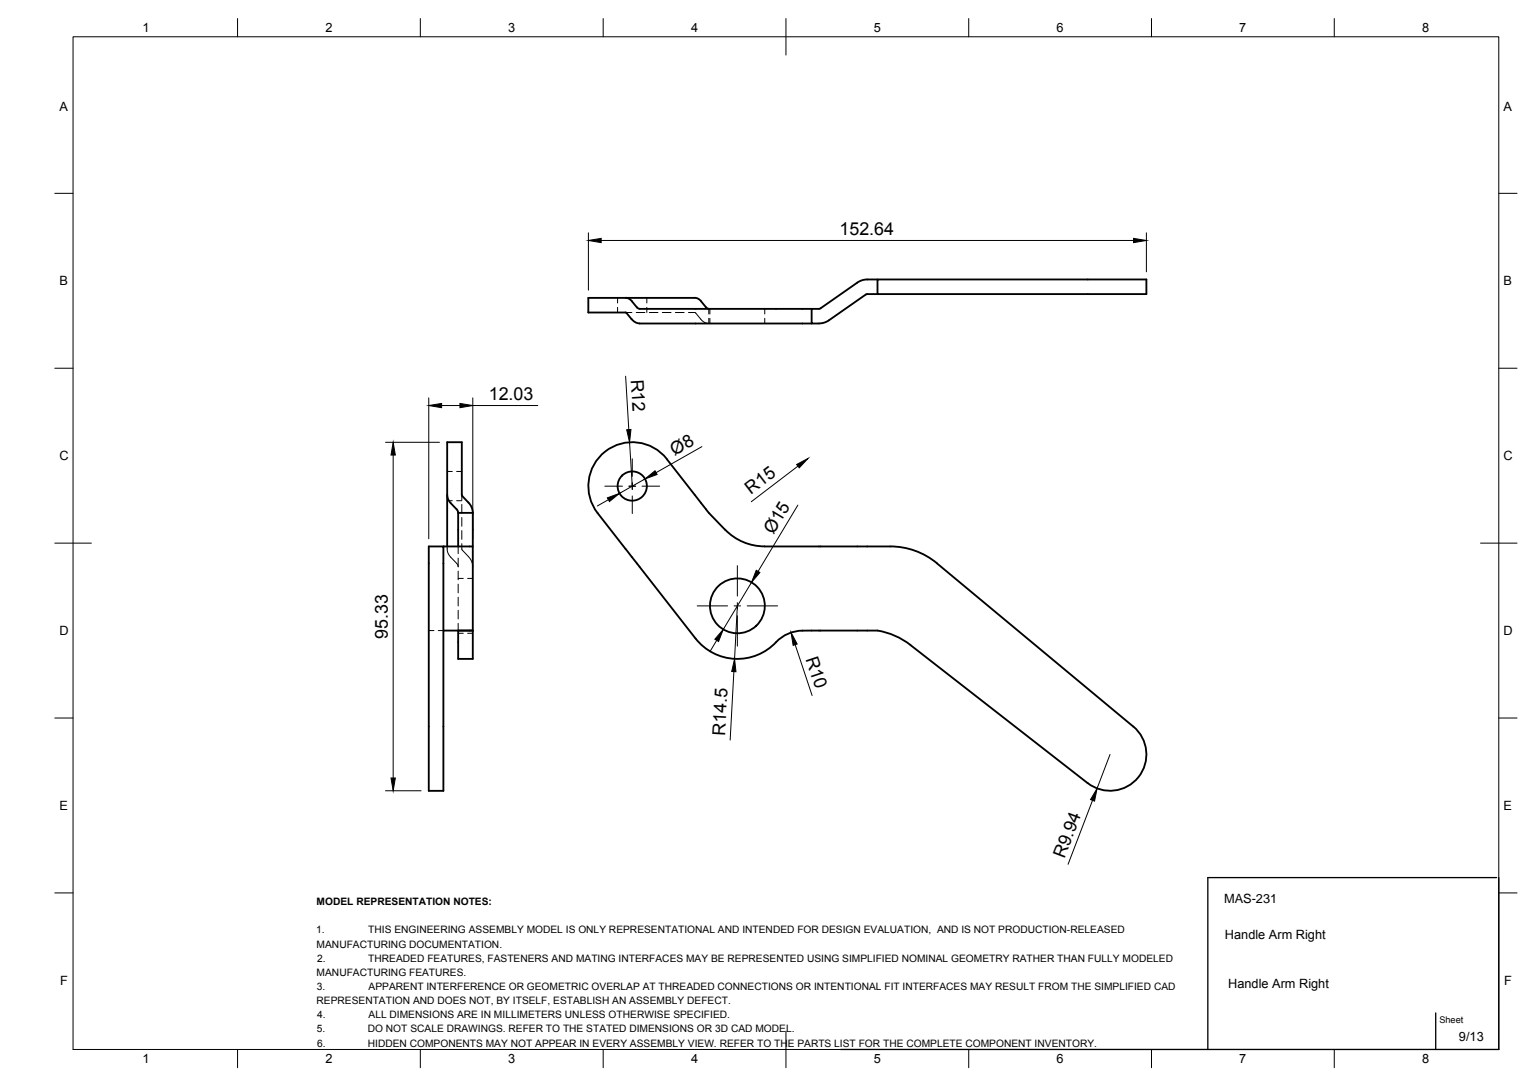
ISO-10303-21;
HEADER;
FILE_DESCRIPTION (('STEP AP214'),
    '1' );
FILE_NAME ( 'Handle Arm Right.step', '2026-10-04T02:08:54', ( '' ), ( '' ), 'STEP AP214', 'Unspecified', '' );
FILE_SCHEMA (( 'AUTOMOTIVE_DESIGN' ));
ENDSEC;
DATA;
#96=CARTESIAN_POINT ( 'NONE',  ( 0.3108999017613323090, 0.9251089822459528378, -1.060267534067256046 ) ) ;
#148=DIRECTION ( 'NONE',  ( -1.000000000000000000, 0.000000000000000000, 0.000000000000000000 ) ) ;
#150=ORIENTED_EDGE ( 'NONE', *, *, #2837, .F. ) ;
#154=DIRECTION ( 'NONE',  ( -1.000000000000000000, -1.802250327717385127E-14, 1.473544972410982106E-14 ) ) ;
#160=DIRECTION ( 'NONE',  ( 0.8191520442889949072, -0.4519843998600416302, 0.3531289150159167556 ) ) ;
#183=VERTEX_POINT ( 'NONE', #42256 ) ;
#188=VECTOR ( 'NONE', #38666, 39.37007874015748143 ) ;
#232=CARTESIAN_POINT ( 'NONE',  ( 0.3161444924769701292, 2.177585298233984279, -3.731703755406948986 ) ) ;
#267=VECTOR ( 'NONE', #18707, 39.37007874015748143 ) ;
#305=CARTESIAN_POINT ( 'NONE',  ( 0.1574803149606299191, 0.5360961046428496246, -0.7563373642699310340 ) ) ;
#307=AXIS2_PLACEMENT_3D ( 'NONE', #8881, #45755, #23738 ) ;
#333=DIRECTION ( 'NONE',  ( 1.000000000000000000, 2.891205793294678326E-16, 0.000000000000000000 ) ) ;
#432=FILL_AREA_STYLE_COLOUR ( '', #44690 ) ;
#457=CARTESIAN_POINT ( 'NONE',  ( 0.2759478392031653460, -0.09842519685039370636, 2.185526306663015728 ) ) ;
#475=DIRECTION ( 'NONE',  ( 0.5735764363510417185, 0.6455006197386566891, -0.5043203561029927506 ) ) ;
#563=CARTESIAN_POINT ( 'NONE',  ( 0.2759478392031586291, -3.539702385322740129E-16, 1.224299699984019663 ) ) ;
#580=VERTEX_POINT ( 'NONE', #5172 ) ;
#606=CARTESIAN_POINT ( 'NONE',  ( 0.1574803149606299191, 0.6241017553149685870, 0.3240160679609070948 ) ) ;
#622=CYLINDRICAL_SURFACE ( 'NONE', #2285, 0.1574803149606297803 ) ;
#656=DIRECTION ( 'NONE',  ( -1.000000000000000000, 0.000000000000000000, 7.051687499798870116E-15 ) ) ;
#688=ORIENTED_EDGE ( 'NONE', *, *, #3021, .T. ) ;
#710=ORIENTED_EDGE ( 'NONE', *, *, #12023, .T. ) ;
#712=VERTEX_POINT ( 'NONE', #45900 ) ;
#730=ADVANCED_FACE ( 'NONE', ( #7834 ), #25829, .F. ) ;
#732=DIRECTION ( 'NONE',  ( 0.000000000000000000, -0.7880107536067199048, 0.6156614753256609562 ) ) ;
#801=CARTESIAN_POINT ( 'NONE',  ( 0.1627249056762492263, 1.099487083487564965, -0.04739565599252298922 ) ) ;
#842=DIRECTION ( 'NONE',  ( 0.7986355100472960489, 0.000000000000000000, -0.6018150231520441595 ) ) ;
#890=ORIENTED_EDGE ( 'NONE', *, *, #19656, .T. ) ;
#907=DIRECTION ( 'NONE',  ( 0.8191520442889899112, -0.4519843998600478474, 0.3531289150159199197 ) ) ;
#943=DIRECTION ( 'NONE',  ( -0.8191520442889950182, 0.4519843998600410750, -0.3531289150159169776 ) ) ;
#974=CIRCLE ( 'NONE', #3327, 0.5708661417322835607 ) ;
#1013=CYLINDRICAL_SURFACE ( 'NONE', #11687, 0.1574803149606297803 ) ;
#1016=CARTESIAN_POINT ( 'NONE',  ( 0.3161444924769291065, 1.914733266569315084, -0.6843357808987579061 ) ) ;
#1036=AXIS2_PLACEMENT_3D ( 'NONE', #44067, #21807, #46957 ) ;
#1075=EDGE_CURVE ( 'NONE', #17962, #28784, #34674, .T. ) ;
#1118=AXIS2_PLACEMENT_3D ( 'NONE', #47069, #18320, #21680 ) ;
#1213=CARTESIAN_POINT ( 'NONE',  ( 0.1574803149606299191, 0.4668427075568346574, -0.7022306805398661478 ) ) ;
#1249=CARTESIAN_POINT ( 'NONE',  ( 0.1574803149606299191, 0.5288907983920094757, -0.7507079620615707549 ) ) ;
#1265=PLANE ( 'NONE',  #18594 ) ;
#1322=FACE_OUTER_BOUND ( 'NONE', #41297, .T. ) ;
#1360=CIRCLE ( 'NONE', #22783, 0.2362204724409449064 ) ;
#1386=CARTESIAN_POINT ( 'NONE',  ( 0.1184675242425283492, -0.5708661417322835607, 1.214596435718460654 ) ) ;
#1400=VECTOR ( 'NONE', #475, 39.37007874015748143 ) ;
#1404=ORIENTED_EDGE ( 'NONE', *, *, #13116, .F. ) ;
#1526=CARTESIAN_POINT ( 'NONE',  ( 0.000000000000000000, 0.6305768042517894134, -0.4926605935704669315 ) ) ;
#1542=LINE ( 'NONE', #23135, #39059 ) ;
#1655=ORIENTED_EDGE ( 'NONE', *, *, #10241, .T. ) ;
#1671=VECTOR ( 'NONE', #1986, 39.37007874015748854 ) ;
#1698=FACE_OUTER_BOUND ( 'NONE', #16346, .T. ) ;
#1743=DIRECTION ( 'NONE',  ( 7.155734338404322954E-15, 0.000000000000000000, 1.000000000000000000 ) ) ;
#1767=VERTEX_POINT ( 'NONE', #2534 ) ;
#1780=VECTOR ( 'NONE', #20781, 39.37007874015748143 ) ;
#1820=DIRECTION ( 'NONE',  ( -5.724375810226263558E-16, -0.6156614753256592909, -0.7880107536067213481 ) ) ;
#1831=CARTESIAN_POINT ( 'NONE',  ( 0.1574803149606299191, 0.3740157480314960647, 1.004692544842683111 ) ) ;
#1839=ORIENTED_EDGE ( 'NONE', *, *, #26366, .T. ) ;
#1843=LINE ( 'NONE', #23903, #35866 ) ;
#1867=ORIENTED_EDGE ( 'NONE', *, *, #8153, .F. ) ;
#1870=CARTESIAN_POINT ( 'NONE',  ( 0.1574803149606299191, 0.4668427075568346574, -0.7022306805398661478 ) ) ;
#1872=DIRECTION ( 'NONE',  ( 1.000000000000000000, 0.000000000000000000, 0.000000000000000000 ) ) ;
#1903=ADVANCED_FACE ( 'NONE', ( #8262 ), #36341, .T. ) ;
#1912=LINE ( 'NONE', #35237, #37906 ) ;
#1986=DIRECTION ( 'NONE',  ( 0.000000000000000000, 0.7880107536067212370, -0.6156614753256591799 ) ) ;
#1997=CARTESIAN_POINT ( 'NONE',  ( 0.4736248074375440931, 1.890321945096787193, -4.194630839571732217 ) ) ;
#2053=CARTESIAN_POINT ( 'NONE',  ( 0.000000000000000000, 0.4666052258408008302, -0.7025346432751023995 ) ) ;
#2057=VERTEX_POINT ( 'NONE', #16188 ) ;
#2085=ORIENTED_EDGE ( 'NONE', *, *, #38033, .T. ) ;
#2127=ORIENTED_EDGE ( 'NONE', *, *, #36636, .T. ) ;
#2131=CYLINDRICAL_SURFACE ( 'NONE', #6486, 0.3912448816427545051 ) ;
#2137=CYLINDRICAL_SURFACE ( 'NONE', #29140, 0.07874015748031498729 ) ;
#2139=CARTESIAN_POINT ( 'NONE',  ( 0.1574803149606299191, 1.086379535891623949, -0.03715491745706125948 ) ) ;
#2146=EDGE_CURVE ( 'NONE', #36896, #18734, #9944, .T. ) ;
#2162=EDGE_CURVE ( 'NONE', #18566, #33555, #16421, .T. ) ;
#2164=DIRECTION ( 'NONE',  ( 7.051687499798870116E-15, 0.000000000000000000, 1.000000000000000000 ) ) ;
#2197=VERTEX_POINT ( 'NONE', #4657 ) ;
#2230=AXIS2_PLACEMENT_3D ( 'NONE', #33648, #41237, #4840 ) ;
#2255=DIRECTION ( 'NONE',  ( 1.109243974507663983E-29, 1.000000000000000000, 2.355041373848515369E-15 ) ) ;
#2285=AXIS2_PLACEMENT_3D ( 'NONE', #44710, #29474, #29932 ) ;
#2368=VECTOR ( 'NONE', #43957, 39.37007874015748854 ) ;
#2426=DIRECTION ( 'NONE',  ( 5.724375810226264544E-16, 0.6156614753256587358, 0.7880107536067215701 ) ) ;
#2515=CARTESIAN_POINT ( 'NONE',  ( 0.3161444924769165610, 1.798092712879858279, -3.826876940038417718 ) ) ;
#2525=AXIS2_PLACEMENT_3D ( 'NONE', #19014, #29636, #37478 ) ;
#2534=CARTESIAN_POINT ( 'NONE',  ( 0.1574803149606299191, 0.4666052258408008302, -0.7025346432751023995 ) ) ;
#2537=ORIENTED_EDGE ( 'NONE', *, *, #20684, .T. ) ;
#2566=DIRECTION ( 'NONE',  ( -3.769839275579535403E-17, 0.7880107536067207930, -0.6156614753256599570 ) ) ;
#2570=CARTESIAN_POINT ( 'NONE',  ( 0.3161444924769519216, 1.488499961090669288, -0.3513258257898460579 ) ) ;
#2588=ORIENTED_EDGE ( 'NONE', *, *, #47395, .F. ) ;
#2603=MECHANICAL_DESIGN_GEOMETRIC_PRESENTATION_REPRESENTATION('',(#12604),#30958);
#2604=DIRECTION ( 'NONE',  ( 1.000000000000000000, 0.000000000000000000, 0.000000000000000000 ) ) ;
#2675=DIRECTION ( 'NONE',  ( -1.000000000000000000, 5.464378949326940770E-15, -4.275490733183370330E-15 ) ) ;
#2683=VECTOR ( 'NONE', #9528, 39.37007874015748854 ) ;
#2700=CARTESIAN_POINT ( 'NONE',  ( 0.4399002236966062518, 0.8539303365987028771, -1.004656681308842447 ) ) ;
#2715=ORIENTED_EDGE ( 'NONE', *, *, #40441, .T. ) ;
#2761=ORIENTED_EDGE ( 'NONE', *, *, #28717, .F. ) ;
#2806=DIRECTION ( 'NONE',  ( 0.000000000000000000, -0.7880107536067206819, 0.6156614753256598460 ) ) ;
#2831=CARTESIAN_POINT ( 'NONE',  ( 0.1126279540338996077, -0.5708661417322835607, 1.206847064312610129 ) ) ;
#2837=EDGE_CURVE ( 'NONE', #24150, #15113, #31611, .T. ) ;
#2918=CARTESIAN_POINT ( 'NONE',  ( 0.3161444924769535869, 1.690605217543005745, -0.5092277576975102749 ) ) ;
#2936=UNCERTAINTY_MEASURE_WITH_UNIT (LENGTH_MEASURE( 1.000000000000000082E-05 ), #19423, 'distance_accuracy_value', 'NONE') ;
#2944=EDGE_LOOP ( 'NONE', ( #31065, #44061, #24696, #6082 ) ) ;
#2955=LINE ( 'NONE', #43213, #5714 ) ;
#2989=EDGE_LOOP ( 'NONE', ( #22664, #46106, #42101, #21732 ) ) ;
#3005=CIRCLE ( 'NONE', #2230, 0.2362204724409449064 ) ;
#3021=EDGE_CURVE ( 'NONE', #7776, #30501, #22148, .T. ) ;
#3044=ORIENTED_EDGE ( 'NONE', *, *, #24684, .T. ) ;
#3053=EDGE_CURVE ( 'NONE', #36104, #36896, #36781, .T. ) ;
#3055=EDGE_LOOP ( 'NONE', ( #8748, #27707, #12776, #33393, #5370, #22939, #8609, #37631, #5677, #29321, #36750, #3117 ) ) ;
#3117=ORIENTED_EDGE ( 'NONE', *, *, #33699, .F. ) ;
#3135=ORIENTED_EDGE ( 'NONE', *, *, #11426, .T. ) ;
#3173=ORIENTED_EDGE ( 'NONE', *, *, #15768, .T. ) ;
#3241=ORIENTED_EDGE ( 'NONE', *, *, #7301, .T. ) ;
#3327=AXIS2_PLACEMENT_3D ( 'NONE', #20136, #12966, #17479 ) ;
#3369=ORIENTED_EDGE ( 'NONE', *, *, #29054, .T. ) ;
#3463=CARTESIAN_POINT ( 'NONE',  ( 0.2759478392031617933, -0.09842519685039370636, 1.713085361781127913 ) ) ;
#3493=CIRCLE ( 'NONE', #30313, 0.3937007874015747699 ) ;
#3515=DIRECTION ( 'NONE',  ( 0.000000000000000000, 2.355041373848520102E-15, -1.000000000000000000 ) ) ;
#3551=CARTESIAN_POINT ( 'NONE',  ( 0.1184675242425281411, 0.3740157480314960647, 1.224299699984021661 ) ) ;
#3566=CARTESIAN_POINT ( 'NONE',  ( 0.2442368959035201015, -0.5708661417322835607, 1.119822416324439018 ) ) ;
#3572=ORIENTED_EDGE ( 'NONE', *, *, #45147, .T. ) ;
#3575=ADVANCED_FACE ( 'NONE', ( #38939 ), #43233, .F. ) ;
#3706=AXIS2_PLACEMENT_3D ( 'NONE', #42837, #2604, #10047 ) ;
#3797=AXIS2_PLACEMENT_3D ( 'NONE', #37657, #19436, #732 ) ;
#3803=CARTESIAN_POINT ( 'NONE',  ( 0.1184675242425198838, 0.000000000000000000, -8.353959598330964227E-16 ) ) ;
#3820=FACE_OUTER_BOUND ( 'NONE', #2989, .T. ) ;
#3827=DIRECTION ( 'NONE',  ( 0.000000000000000000, -1.000000000000000000, 0.000000000000000000 ) ) ;
#3830=ORIENTED_EDGE ( 'NONE', *, *, #41683, .T. ) ;
#3851=EDGE_LOOP ( 'NONE', ( #30997, #24195, #8872, #24931 ) ) ;
#3866=AXIS2_PLACEMENT_3D ( 'NONE', #19137, #5003, #15329 ) ;
#3913=DIRECTION ( 'NONE',  ( -5.159318851433039196E-16, -0.6156614753256609562, -0.7880107536067197938 ) ) ;
#3919=ADVANCED_FACE ( 'NONE', ( #25099 ), #31607, .T. ) ;
#3923=DIRECTION ( 'NONE',  ( -2.114720919224289611E-16, 1.000000000000000000, 0.000000000000000000 ) ) ;
#3930=VECTOR ( 'NONE', #23402, 39.37007874015748143 ) ;
#3971=APPLICATION_CONTEXT ( 'automotive_design' ) ;
#3980=LINE ( 'NONE', #606, #11849 ) ;
#4054=DIRECTION ( 'NONE',  ( 7.047314121155781188E-15, 0.000000000000000000, 1.000000000000000000 ) ) ;
#4143=DIRECTION ( 'NONE',  ( -1.000000000000000000, 0.000000000000000000, -7.051687499798870116E-15 ) ) ;
#4164=DIRECTION ( 'NONE',  ( -5.298843091159153171E-15, -2.355041373848512214E-15, 1.000000000000000000 ) ) ;
#4180=VERTEX_POINT ( 'NONE', #43155 ) ;
#4190=VECTOR ( 'NONE', #3913, 39.37007874015748143 ) ;
#4197=ORIENTED_EDGE ( 'NONE', *, *, #32553, .F. ) ;
#4223=CARTESIAN_POINT ( 'NONE',  ( 0.02847999302535491814, 0.6072747502901004735, -0.8119482170283445210 ) ) ;
#4250=EDGE_CURVE ( 'NONE', #712, #6130, #37711, .T. ) ;
#4273=CARTESIAN_POINT ( 'NONE',  ( 0.4736248074375630224, 0.4457451269443653552, -1.671447902550338815 ) ) ;
#4317=CARTESIAN_POINT ( 'NONE',  ( 0.1864803149606299171, 1.086379535891623949, -0.03715491745706173132 ) ) ;
#4384=DIRECTION ( 'NONE',  ( 0.000000000000000000, -0.6156614753256598460, -0.7880107536067206819 ) ) ;
#4416=ORIENTED_EDGE ( 'NONE', *, *, #40562, .F. ) ;
#4445=EDGE_LOOP ( 'NONE', ( #3241, #15111, #25556, #32618 ) ) ;
#4448=PLANE ( 'NONE',  #30350 ) ;
#4454=EDGE_LOOP ( 'NONE', ( #30362, #10226, #35204, #29981 ) ) ;
#4469=DIRECTION ( 'NONE',  ( -1.000000000000000000, 0.000000000000000000, 0.000000000000000000 ) ) ;
#4470=EDGE_CURVE ( 'NONE', #32150, #42931, #18249, .T. ) ;
#4527=VECTOR ( 'NONE', #17737, 39.37007874015748143 ) ;
#4531=EDGE_LOOP ( 'NONE', ( #18099, #28878, #35700, #13225 ) ) ;
#4543=EDGE_CURVE ( 'NONE', #27121, #2057, #46998, .T. ) ;
#4625=CARTESIAN_POINT ( 'NONE',  ( 0.1184675242425078795, -0.09842519685039370636, 1.713085361781127913 ) ) ;
#4657=CARTESIAN_POINT ( 'NONE',  ( 2.048885995248196921E-16, -0.5708661417322835607, 0.9783464566929134243 ) ) ;
#4663=DIRECTION ( 'NONE',  ( -4.275490733183370330E-15, 0.000000000000000000, 1.000000000000000000 ) ) ;
#4725=CARTESIAN_POINT ( 'NONE',  ( 0.000000000000000000, 3.616083068348484413E-17, -0.2952755905511810774 ) ) ;
#4741=LINE ( 'NONE', #33791, #6344 ) ;
#4755=AXIS2_PLACEMENT_3D ( 'NONE', #5649, #20260, #6102 ) ;
#4767=ORIENTED_EDGE ( 'NONE', *, *, #18776, .T. ) ;
#4840=DIRECTION ( 'NONE',  ( 1.000000000000000000, 2.891205793294678326E-16, 0.000000000000000000 ) ) ;
#4880=MANIFOLD_SOLID_BREP ( 'Handle Arm Right', #31751 ) ;
#4924=PLANE ( 'NONE',  #29481 ) ;
#4948=AXIS2_PLACEMENT_3D ( 'NONE', #23717, #5496, #30694 ) ;
#4958=CARTESIAN_POINT ( 'NONE',  ( 0.2759478392031653460, 0.3740157480314960647, 2.185526306663015728 ) ) ;
#4972=ADVANCED_FACE ( 'NONE', ( #36875, #11476 ), #40211, .T. ) ;
#5003=DIRECTION ( 'NONE',  ( 5.724375810226257641E-16, 0.6156614753256588468, 0.7880107536067216811 ) ) ;
#5082=FACE_OUTER_BOUND ( 'NONE', #14954, .T. ) ;
#5117=ORIENTED_EDGE ( 'NONE', *, *, #23549, .T. ) ;
#5144=CARTESIAN_POINT ( 'NONE',  ( 0.1184675242425078795, -0.09842519685039370636, 1.713085361781127913 ) ) ;
#5172=CARTESIAN_POINT ( 'NONE',  ( 0.4736248074375835060, 1.690605217543005745, -0.5092277576975118292 ) ) ;
#5237=DIRECTION ( 'NONE',  ( -5.464378949326941559E-15, -1.000000000000000000, 0.000000000000000000 ) ) ;
#5247=ORIENTED_EDGE ( 'NONE', *, *, #4250, .T. ) ;
#5343=CARTESIAN_POINT ( 'NONE',  ( 0.03372458374097370148, 0.6131769916352027838, -0.8165595533554468322 ) ) ;
#5367=CARTESIAN_POINT ( 'NONE',  ( 0.1733357866104494327, -0.5708661417322835607, 1.025733466389925352 ) ) ;
#5370=ORIENTED_EDGE ( 'NONE', *, *, #44949, .F. ) ;
#5378=FACE_OUTER_BOUND ( 'NONE', #29897, .T. ) ;
#5401=AXIS2_PLACEMENT_3D ( 'NONE', #42962, #13754, #6791 ) ;
#5403=CARTESIAN_POINT ( 'NONE',  ( 0.4736248074375433714, 2.559880088878740079, -3.648497683167389649 ) ) ;
#5446=VECTOR ( 'NONE', #41680, 39.37007874015748143 ) ;
#5465=DIRECTION ( 'NONE',  ( -1.000000000000000000, -1.413024824309076326E-14, 1.884033099078770012E-14 ) ) ;
#5479=CIRCLE ( 'NONE', #39127, 0.3912448816427545051 ) ;
#5496=DIRECTION ( 'NONE',  ( 4.190354514309263844E-15, -0.9699617890481126992, -0.2432573283306889433 ) ) ;
#5536=ADVANCED_BREP_SHAPE_REPRESENTATION ( 'Handle Arm Right', ( #4880, #20860 ), #27025 ) ;
#5540=DIRECTION ( 'NONE',  ( 0.000000000000000000, 2.355041373848520102E-15, -1.000000000000000000 ) ) ;
#5563=FACE_OUTER_BOUND ( 'NONE', #13406, .T. ) ;
#5570=ADVANCED_FACE ( 'NONE', ( #20635, #41946 ), #39074, .F. ) ;
#5584=DIRECTION ( 'NONE',  ( -1.000000000000000000, 0.000000000000000000, 7.155734338404321376E-15 ) ) ;
#5625=CIRCLE ( 'NONE', #2525, 0.4724409448818896462 ) ;
#5626=VERTEX_POINT ( 'NONE', #28572 ) ;
#5649=CARTESIAN_POINT ( 'NONE',  ( 0.1864803149606299171, 1.086379535891623949, -0.03715491745706165500 ) ) ;
#5673=ORIENTED_EDGE ( 'NONE', *, *, #42018, .F. ) ;
#5677=ORIENTED_EDGE ( 'NONE', *, *, #17755, .F. ) ;
#5708=PLANE ( 'NONE',  #6732 ) ;
#5714=VECTOR ( 'NONE', #13761, 39.37007874015748854 ) ;
#5748=ADVANCED_FACE ( 'NONE', ( #11772 ), #37375, .T. ) ;
#5862=EDGE_CURVE ( 'NONE', #18361, #8850, #42608, .T. ) ;
#5864=VERTEX_POINT ( 'NONE', #2139 ) ;
#5962=AXIS2_PLACEMENT_3D ( 'NONE', #40068, #25952, #17812 ) ;
#5964=CARTESIAN_POINT ( 'NONE',  ( 0.2362204724409449064, -0.5708661417322835607, 0.9783464566929134243 ) ) ;
#5979=CIRCLE ( 'NONE', #45788, 0.4724409448818899238 ) ;
#6019=CARTESIAN_POINT ( 'NONE',  ( 0.2871444924769520068, 1.495705267341507883, -0.3569552279982047271 ) ) ;
#6035=DIRECTION ( 'NONE',  ( 0.000000000000000000, -1.000000000000000000, 0.000000000000000000 ) ) ;
#6082=ORIENTED_EDGE ( 'NONE', *, *, #34470, .F. ) ;
#6102=DIRECTION ( 'NONE',  ( -0.8191520442889957954, 0.4519843998600397428, -0.3531289150159173662 ) ) ;
#6130=VERTEX_POINT ( 'NONE', #25072 ) ;
#6254=ORIENTED_EDGE ( 'NONE', *, *, #27428, .T. ) ;
#6306=VERTEX_POINT ( 'NONE', #33949 ) ;
#6324=DIRECTION ( 'NONE',  ( -1.000000000000000000, 0.000000000000000000, 0.000000000000000000 ) ) ;
#6326=ADVANCED_FACE ( 'NONE', ( #20474 ), #13302, .T. ) ;
#6344=VECTOR ( 'NONE', #907, 39.37007874015748854 ) ;
#6404=DIRECTION ( 'NONE',  ( -1.000000000000000000, 0.000000000000000000, 0.000000000000000000 ) ) ;
#6428=EDGE_CURVE ( 'NONE', #11697, #44566, #23137, .T. ) ;
#6464=CARTESIAN_POINT ( 'NONE',  ( 0.1627249056762490320, 0.5419983459879528231, -0.7609487005970335671 ) ) ;
#6486=AXIS2_PLACEMENT_3D ( 'NONE', #16302, #30930, #31162 ) ;
#6525=ORIENTED_EDGE ( 'NONE', *, *, #8153, .T. ) ;
#6535=FACE_OUTER_BOUND ( 'NONE', #33407, .T. ) ;
#6567=AXIS2_PLACEMENT_3D ( 'NONE', #25527, #6324, #31990 ) ;
#6621=ORIENTED_EDGE ( 'NONE', *, *, #38033, .F. ) ;
#6626=CARTESIAN_POINT ( 'NONE',  ( 0.03372458374097409700, 1.170665729134817035, -0.1030065087509350469 ) ) ;
#6643=AXIS2_PLACEMENT_3D ( 'NONE', #1249, #38393, #30994 ) ;
#6673=LINE ( 'NONE', #18411, #8818 ) ;
#6704=ORIENTED_EDGE ( 'NONE', *, *, #26274, .T. ) ;
#6732=AXIS2_PLACEMENT_3D ( 'NONE', #1386, #16044, #1872 ) ;
#6746=FACE_OUTER_BOUND ( 'NONE', #18691, .T. ) ;
#6751=CARTESIAN_POINT ( 'NONE',  ( 0.3108999017613326976, 1.482597719745565090, -0.3467144894627433027 ) ) ;
#6765=DIRECTION ( 'NONE',  ( 0.000000000000000000, -0.9945218953682737340, -0.1045284632676499736 ) ) ;
#6771=DIRECTION ( 'NONE',  ( 5.724375810226260600E-16, 0.6156614753256579586, 0.7880107536067221252 ) ) ;
#6791=DIRECTION ( 'NONE',  ( 0.000000000000000000, 0.000000000000000000, -1.000000000000000000 ) ) ;
#6792=LINE ( 'NONE', #305, #41989 ) ;
#6797=ORIENTED_EDGE ( 'NONE', *, *, #2837, .T. ) ;
#6835=CARTESIAN_POINT ( 'NONE',  ( 0.1184675242425066999, -0.09842519685039370636, 1.870565676741756000 ) ) ;
#6879=CARTESIAN_POINT ( 'NONE',  ( 0.1574803149606299191, 1.086379535891623949, -0.03715491745706125948 ) ) ;
#6920=ADVANCED_FACE ( 'NONE', ( #40151 ), #10724, .F. ) ;
#6930=CARTESIAN_POINT ( 'NONE',  ( 0.1574803149606299191, 0.3883517482604913473, -0.6419475548153091848 ) ) ;
#6949=FACE_OUTER_BOUND ( 'NONE', #21995, .T. ) ;
#6959=DIRECTION ( 'NONE',  ( -5.411399086424348811E-15, -1.000000000000000000, 0.000000000000000000 ) ) ;
#6993=CARTESIAN_POINT ( 'NONE',  ( 0.1574803149606299191, -0.5708661417322835607, -6.991093932140394160E-17 ) ) ;
#7036=EDGE_CURVE ( 'NONE', #28784, #17791, #7994, .T. ) ;
#7080=LINE ( 'NONE', #32026, #16132 ) ;
#7168=LENGTH_MEASURE_WITH_UNIT ( LENGTH_MEASURE( 0.02539999999999999897 ), #44051 ) ;
#7193=CYLINDRICAL_SURFACE ( 'NONE', #46643, 0.4724409448818896462 ) ;
#7221=ORIENTED_EDGE ( 'NONE', *, *, #39267, .T. ) ;
#7222=ORIENTED_EDGE ( 'NONE', *, *, #19756, .T. ) ;
#7223=AXIS2_PLACEMENT_3D ( 'NONE', #38987, #28723, #42791 ) ;
#7249=FACE_OUTER_BOUND ( 'NONE', #42234, .T. ) ;
#7300=CARTESIAN_POINT ( 'NONE',  ( 0.2362204724409449064, -0.5708661417322835607, 0.9783464566929134243 ) ) ;
#7301=EDGE_CURVE ( 'NONE', #28693, #580, #2955, .T. ) ;
#7321=ADVANCED_FACE ( 'NONE', ( #39153 ), #25023, .F. ) ;
#7418=DIRECTION ( 'NONE',  ( -1.000000000000000000, -5.377642775528100415E-15, 4.197754538034199640E-15 ) ) ;
#7515=AXIS2_PLACEMENT_3D ( 'NONE', #24865, #36130, #25356 ) ;
#7522=CARTESIAN_POINT ( 'NONE',  ( 0.1627249056762490320, 0.5419983459879528231, -0.7609487005970335671 ) ) ;
#7525=DIRECTION ( 'NONE',  ( -1.000000000000000000, 0.000000000000000000, -7.047314121155770932E-15 ) ) ;
#7535=EDGE_CURVE ( 'NONE', #5864, #18566, #12069, .T. ) ;
#7572=FACE_OUTER_BOUND ( 'NONE', #9048, .T. ) ;
#7583=DIRECTION ( 'NONE',  ( 0.000000000000000000, 0.000000000000000000, -1.000000000000000000 ) ) ;
#7601=ORIENTED_EDGE ( 'NONE', *, *, #7616, .F. ) ;
#7616=EDGE_CURVE ( 'NONE', #12883, #35279, #40554, .T. ) ;
#7656=ORIENTED_EDGE ( 'NONE', *, *, #19032, .F. ) ;
#7672=ORIENTED_EDGE ( 'NONE', *, *, #7301, .F. ) ;
#7673=CARTESIAN_POINT ( 'NONE',  ( 0.2871444924769515628, 0.9382165298418956301, -1.070508272602716637 ) ) ;
#7678=EDGE_LOOP ( 'NONE', ( #19026, #15942, #11771, #16125 ) ) ;
#7704=VERTEX_POINT ( 'NONE', #19473 ) ;
#7774=LINE ( 'NONE', #22152, #32248 ) ;
#7776=VERTEX_POINT ( 'NONE', #44312 ) ;
#7819=CARTESIAN_POINT ( 'NONE',  ( 0.08946752424252854552, 0.3740157480314960647, 1.224299699984021661 ) ) ;
#7824=CARTESIAN_POINT ( 'NONE',  ( 0.1574803149606299191, 0.000000000000000000, 0.000000000000000000 ) ) ;
#7834=FACE_OUTER_BOUND ( 'NONE', #4531, .T. ) ;
#7867=SURFACE_STYLE_FILL_AREA ( #22017 ) ;
#7896=CIRCLE ( 'NONE', #30780, 0.1574803149606300579 ) ;
#7915=DIRECTION ( 'NONE',  ( 1.000000000000000000, -5.859809909139239229E-15, 3.662381193212024616E-15 ) ) ;
#7951=EDGE_CURVE ( 'NONE', #36924, #39408, #38568, .T. ) ;
#7976=ORIENTED_EDGE ( 'NONE', *, *, #46184, .T. ) ;
#7994=CIRCLE ( 'NONE', #14134, 0.07874015748031495954 ) ;
#8016=ADVANCED_FACE ( 'NONE', ( #8857 ), #16069, .T. ) ;
#8039=ADVANCED_FACE ( 'NONE', ( #23961 ), #2131, .T. ) ;
#8123=DIRECTION ( 'NONE',  ( 7.888609052210116302E-31, 0.6156614753256598460, 0.7880107536067206819 ) ) ;
#8153=EDGE_CURVE ( 'NONE', #8512, #8746, #32996, .T. ) ;
#8157=ORIENTED_EDGE ( 'NONE', *, *, #42018, .T. ) ;
#8186=FACE_OUTER_BOUND ( 'NONE', #42368, .T. ) ;
#8237=LINE ( 'NONE', #22628, #25525 ) ;
#8262=FACE_OUTER_BOUND ( 'NONE', #7678, .T. ) ;
#8272=ORIENTED_EDGE ( 'NONE', *, *, #20714, .F. ) ;
#8352=AXIS2_PLACEMENT_3D ( 'NONE', #47298, #14475, #11126 ) ;
#8418=ORIENTED_EDGE ( 'NONE', *, *, #25778, .F. ) ;
#8431=ORIENTED_EDGE ( 'NONE', *, *, #47080, .F. ) ;
#8442=CARTESIAN_POINT ( 'NONE',  ( 0.4736248074375795647, 1.205832402325950792, -1.129708666049259902 ) ) ;
#8446=DIRECTION ( 'NONE',  ( 0.000000000000000000, 0.7880107536067221252, -0.6156614753256580697 ) ) ;
#8447=VERTEX_POINT ( 'NONE', #32881 ) ;
#8460=DIRECTION ( 'NONE',  ( -0.7986355100472960489, 0.000000000000000000, 0.6018150231520440485 ) ) ;
#8462=CARTESIAN_POINT ( 'NONE',  ( 0.1184675242425285574, -0.5708661417322835607, 1.224299699984021661 ) ) ;
#8508=CARTESIAN_POINT ( 'NONE',  ( 0.3161444924769519216, 0.9382165298418937427, -1.070508272602716637 ) ) ;
#8512=VERTEX_POINT ( 'NONE', #8626 ) ;
#8520=AXIS2_PLACEMENT_3D ( 'NONE', #24172, #34958, #42355 ) ;
#8556=EDGE_CURVE ( 'NONE', #11697, #9878, #36385, .T. ) ;
#8609=ORIENTED_EDGE ( 'NONE', *, *, #16733, .F. ) ;
#8626=CARTESIAN_POINT ( 'NONE',  ( 0.1126279540338993995, 0.3740157480314960647, 1.206847064312612128 ) ) ;
#8703=LINE ( 'NONE', #8462, #27944 ) ;
#8708=EDGE_CURVE ( 'NONE', #19538, #42619, #1912, .T. ) ;
#8746=VERTEX_POINT ( 'NONE', #2831 ) ;
#8748=ORIENTED_EDGE ( 'NONE', *, *, #20509, .T. ) ;
#8766=CARTESIAN_POINT ( 'NONE',  ( 0.4736248074375590811, 1.914733266569315084, -0.6843357808987579061 ) ) ;
#8806=ORIENTED_EDGE ( 'NONE', *, *, #10241, .F. ) ;
#8818=VECTOR ( 'NONE', #22006, 39.37007874015748854 ) ;
#8829=FACE_OUTER_BOUND ( 'NONE', #38501, .T. ) ;
#8850=VERTEX_POINT ( 'NONE', #24666 ) ;
#8857=FACE_OUTER_BOUND ( 'NONE', #43000, .T. ) ;
#8872=ORIENTED_EDGE ( 'NONE', *, *, #47295, .T. ) ;
#8881=CARTESIAN_POINT ( 'NONE',  ( 0.1184675242425320824, -0.09842519685039370636, 1.713085361781127913 ) ) ;
#8900=EDGE_LOOP ( 'NONE', ( #43755, #36739, #4767, #8272 ) ) ;
#8928=PLANE ( 'NONE',  #6643 ) ;
#8935=EDGE_CURVE ( 'NONE', #18734, #28644, #6673, .T. ) ;
#8961=DIRECTION ( 'NONE',  ( -0.8191520442889947962, 0.4519843998600418522, -0.3531289150159164225 ) ) ;
#9048=EDGE_LOOP ( 'NONE', ( #24849, #890, #35106, #43245 ) ) ;
#9145=CARTESIAN_POINT ( 'NONE',  ( 0.1574803149606299191, 3.616083068348484413E-17, -0.2952755905511810774 ) ) ;
#9150=EDGE_CURVE ( 'NONE', #34943, #15113, #36409, .T. ) ;
#9226=ORIENTED_EDGE ( 'NONE', *, *, #22462, .T. ) ;
#9228=CARTESIAN_POINT ( 'NONE',  ( 0.08946752424252873981, -0.5708661417322835607, 1.224299699984019663 ) ) ;
#9252=CARTESIAN_POINT ( 'NONE',  ( 0.4736248074375590811, 1.914733266569315084, -0.6843357808987579061 ) ) ;
#9268=CARTESIAN_POINT ( 'NONE',  ( 0.2759478392031586291, -0.5708661417322835607, 1.224299699984019663 ) ) ;
#9281=VECTOR ( 'NONE', #45470, 39.37007874015748143 ) ;
#9283=LINE ( 'NONE', #4958, #22201 ) ;
#9323=ADVANCED_FACE ( 'NONE', ( #5563 ), #20414, .F. ) ;
#9333=VECTOR ( 'NONE', #19848, 39.37007874015748143 ) ;
#9335=SHAPE_REPRESENTATION ( 'Handle Arm Right', ( #20860 ), #27025 ) ;
#9368=EDGE_CURVE ( 'NONE', #35620, #42894, #38630, .T. ) ;
#9471=ORIENTED_EDGE ( 'NONE', *, *, #5862, .F. ) ;
#9485=ADVANCED_FACE ( 'NONE', ( #41477 ), #8928, .T. ) ;
#9528=DIRECTION ( 'NONE',  ( -1.665334536937734071E-16, -0.6156614753256598460, -0.7880107536067206819 ) ) ;
#9548=CARTESIAN_POINT ( 'NONE',  ( 0.000000000000000000, 0.08719492171395729074, -0.5641677032617165022 ) ) ;
#9593=ORIENTED_EDGE ( 'NONE', *, *, #37545, .F. ) ;
#9634=CARTESIAN_POINT ( 'NONE',  ( 0.000000000000000000, -5.122214988120488358E-16, -8.878505979408856939E-16 ) ) ;
#9648=ORIENTED_EDGE ( 'NONE', *, *, #29660, .T. ) ;
#9675=CARTESIAN_POINT ( 'NONE',  ( 0.4736248074375818407, 1.495705267341505884, -0.3569552279982035614 ) ) ;
#9769=CARTESIAN_POINT ( 'NONE',  ( 0.4736248074376000483, 2.177585298233984279, -3.731703755406948986 ) ) ;
#9781=DIRECTION ( 'NONE',  ( 7.155734338404322954E-15, 0.000000000000000000, 1.000000000000000000 ) ) ;
#9782=FACE_BOUND ( 'NONE', #35849, .T. ) ;
#9816=EDGE_CURVE ( 'NONE', #34943, #24486, #47225, .T. ) ;
#9817=VECTOR ( 'NONE', #45261, 39.37007874015748143 ) ;
#9830=EDGE_LOOP ( 'NONE', ( #11499, #41064, #11584, #46993 ) ) ;
#9854=EDGE_CURVE ( 'NONE', #42441, #38536, #40463, .T. ) ;
#9864=ADVANCED_FACE ( 'NONE', ( #6535 ), #31963, .T. ) ;
#9878=VERTEX_POINT ( 'NONE', #11269 ) ;
#9916=ADVANCED_FACE ( 'NONE', ( #3820 ), #46548, .F. ) ;
#9939=VERTEX_POINT ( 'NONE', #33562 ) ;
#9944=CIRCLE ( 'NONE', #16086, 0.02900000000000009515 ) ;
#10047=DIRECTION ( 'NONE',  ( 0.000000000000000000, 0.000000000000000000, -1.000000000000000000 ) ) ;
#10097=ORIENTED_EDGE ( 'NONE', *, *, #19204, .T. ) ;
#10107=DIRECTION ( 'NONE',  ( -2.943801717310650128E-16, 1.000000000000000000, 2.355041373848525230E-15 ) ) ;
#10179=AXIS2_PLACEMENT_3D ( 'NONE', #41044, #19015, #4164 ) ;
#10226=ORIENTED_EDGE ( 'NONE', *, *, #27723, .T. ) ;
#10241=EDGE_CURVE ( 'NONE', #22983, #44566, #24277, .T. ) ;
#10260=CARTESIAN_POINT ( 'NONE',  ( 0.1574803149606299191, -5.122214988120488358E-16, -8.878505979408856939E-16 ) ) ;
#10306=CARTESIAN_POINT ( 'NONE',  ( 0.000000000000000000, -0.5708661417322835607, -6.991093932140394160E-17 ) ) ;
#10396=ORIENTED_EDGE ( 'NONE', *, *, #40796, .T. ) ;
#10419=VERTEX_POINT ( 'NONE', #11397 ) ;
#10457=DIRECTION ( 'NONE',  ( 1.000000000000000000, 1.751623080406019977E-46, -7.049916206369740876E-15 ) ) ;
#10724=PLANE ( 'NONE',  #17174 ) ;
#10764=ORIENTED_EDGE ( 'NONE', *, *, #14364, .T. ) ;
#10788=SURFACE_STYLE_USAGE ( .BOTH. , #40670 ) ;
#10834=ORIENTED_EDGE ( 'NONE', *, *, #22025, .F. ) ;
#10835=DIRECTION ( 'NONE',  ( 1.000000000000000000, 0.000000000000000000, 0.000000000000000000 ) ) ;
#10907=VECTOR ( 'NONE', #42440, 39.37007874015748143 ) ;
#11010=ORIENTED_EDGE ( 'NONE', *, *, #33199, .F. ) ;
#11046=PLANE ( 'NONE',  #47419 ) ;
#11068=ORIENTED_EDGE ( 'NONE', *, *, #35855, .F. ) ;
#11086=LINE ( 'NONE', #27378, #18535 ) ;
#11118=EDGE_CURVE ( 'NONE', #32266, #44909, #39890, .T. ) ;
#11126=DIRECTION ( 'NONE',  ( 0.000000000000000000, -0.7880107536067197938, 0.6156614753256609562 ) ) ;
#11136=VECTOR ( 'NONE', #31000, 39.37007874015748854 ) ;
#11149=LINE ( 'NONE', #11382, #33901 ) ;
#11160=DIRECTION ( 'NONE',  ( 7.051687499798870116E-15, 0.000000000000000000, 1.000000000000000000 ) ) ;
#11184=EDGE_LOOP ( 'NONE', ( #23702, #19395, #18389, #40318, #47287, #19417, #32843, #3044, #23834, #37581, #10764, #16990 ) ) ;
#11213=CARTESIAN_POINT ( 'NONE',  ( 0.03171094329963846520, 0.3740157480314960647, 1.099466564236704746 ) ) ;
#11269=CARTESIAN_POINT ( 'NONE',  ( 0.1574803149606299191, 0.000000000000000000, 0.2952755905511810774 ) ) ;
#11274=FACE_OUTER_BOUND ( 'NONE', #18877, .T. ) ;
#11354=CIRCLE ( 'NONE', #5962, 0.1864803149606299448 ) ;
#11360=ORIENTED_EDGE ( 'NONE', *, *, #36047, .T. ) ;
#11382=CARTESIAN_POINT ( 'NONE',  ( 0.1574803149606299191, 0.4668427075568346574, -0.7022306805398661478 ) ) ;
#11397=CARTESIAN_POINT ( 'NONE',  ( 0.2759478392031630145, -0.09842519685039370636, 1.870565676741759775 ) ) ;
#11426=EDGE_CURVE ( 'NONE', #6306, #40667, #11354, .T. ) ;
#11476=FACE_OUTER_BOUND ( 'NONE', #23551, .T. ) ;
#11499=ORIENTED_EDGE ( 'NONE', *, *, #24906, .T. ) ;
#11576=ORIENTED_EDGE ( 'NONE', *, *, #20913, .T. ) ;
#11584=ORIENTED_EDGE ( 'NONE', *, *, #38703, .F. ) ;
#11588=DIRECTION ( 'NONE',  ( -1.000000000000000000, -5.377642775528100415E-15, 4.197754538034575138E-15 ) ) ;
#11630=ORIENTED_EDGE ( 'NONE', *, *, #6428, .T. ) ;
#11631=LINE ( 'NONE', #29646, #23030 ) ;
#11660=ORIENTED_EDGE ( 'NONE', *, *, #31147, .T. ) ;
#11687=AXIS2_PLACEMENT_3D ( 'NONE', #15905, #44856, #34574 ) ;
#11691=DIRECTION ( 'NONE',  ( 0.000000000000000000, 0.000000000000000000, 1.000000000000000000 ) ) ;
#11697=VERTEX_POINT ( 'NONE', #9145 ) ;
#11771=ORIENTED_EDGE ( 'NONE', *, *, #16427, .T. ) ;
#11772=FACE_OUTER_BOUND ( 'NONE', #29279, .T. ) ;
#11792=EDGE_CURVE ( 'NONE', #24385, #32150, #29722, .T. ) ;
#11849=VECTOR ( 'NONE', #29685, 39.37007874015748854 ) ;
#11903=DIRECTION ( 'NONE',  ( 0.000000000000000000, -1.000000000000000000, 0.000000000000000000 ) ) ;
#11930=DIRECTION ( 'NONE',  ( 5.159318851433039196E-16, 0.6156614753256609562, 0.7880107536067197938 ) ) ;
#11953=AXIS2_PLACEMENT_3D ( 'NONE', #19333, #11930, #33982 ) ;
#11971=CARTESIAN_POINT ( 'NONE',  ( 0.4736248074375614681, 1.025704337919490117, -1.138861239548320858 ) ) ;
#11992=ORIENTED_EDGE ( 'NONE', *, *, #12023, .F. ) ;
#12015=ORIENTED_EDGE ( 'NONE', *, *, #22719, .F. ) ;
#12023=EDGE_CURVE ( 'NONE', #5626, #27121, #18684, .T. ) ;
#12029=FACE_OUTER_BOUND ( 'NONE', #18418, .T. ) ;
#12060=FACE_OUTER_BOUND ( 'NONE', #40547, .T. ) ;
#12066=DIRECTION ( 'NONE',  ( -5.724375810226267502E-16, -0.6156614753256588468, -0.7880107536067216811 ) ) ;
#12069=LINE ( 'NONE', #14715, #4190 ) ;
#12175=DIRECTION ( 'NONE',  ( 1.000000000000000000, 0.000000000000000000, -7.044195017643630340E-15 ) ) ;
#12193=FACE_OUTER_BOUND ( 'NONE', #22167, .T. ) ;
#12368=DIRECTION ( 'NONE',  ( -1.000000000000000000, 5.472378587457090550E-15, -4.275490733183370330E-15 ) ) ;
#12392=LINE ( 'NONE', #8766, #39135 ) ;
#12407=EDGE_LOOP ( 'NONE', ( #20343, #11360, #31214, #36046 ) ) ;
#12430=EDGE_CURVE ( 'NONE', #45189, #36896, #40255, .T. ) ;
#12451=EDGE_LOOP ( 'NONE', ( #7601, #11068, #28752, #2715 ) ) ;
#12479=CARTESIAN_POINT ( 'NONE',  ( 0.1574803149606299191, -0.5708661417322835607, -6.991093932140394160E-17 ) ) ;
#12494=VECTOR ( 'NONE', #36258, 39.37007874015748854 ) ;
#12545=DIRECTION ( 'NONE',  ( 1.000000000000000000, 0.000000000000000000, 0.000000000000000000 ) ) ;
#12549=DIRECTION ( 'NONE',  ( -1.000000000000000000, 0.000000000000000000, 0.000000000000000000 ) ) ;
#12557=SHAPE_DEFINITION_REPRESENTATION ( #40586, #9335 ) ;
#12565=DIRECTION ( 'NONE',  ( 0.000000000000000000, 1.000000000000000000, 2.891205793294680298E-16 ) ) ;
#12572=ORIENTED_EDGE ( 'NONE', *, *, #16561, .T. ) ;
#12604=STYLED_ITEM ( 'NONE', ( #18193 ), #4880 ) ;
#12669=DIRECTION ( 'NONE',  ( 0.000000000000000000, 0.000000000000000000, -1.000000000000000000 ) ) ;
#12738=SHAPE_REPRESENTATION_RELATIONSHIP ( 'NONE' , 'NONE' ,  #9335, #5536 ) ;
#12776=ORIENTED_EDGE ( 'NONE', *, *, #11118, .F. ) ;
#12798=CARTESIAN_POINT ( 'NONE',  ( 0.000000000000000000, -0.1637340966949556997, -0.2095700869694007984 ) ) ;
#12802=PLANE ( 'NONE',  #26908 ) ;
#12819=ORIENTED_EDGE ( 'NONE', *, *, #34372, .T. ) ;
#12883=VERTEX_POINT ( 'NONE', #46685 ) ;
#12892=VECTOR ( 'NONE', #38777, 39.37007874015748143 ) ;
#12898=LINE ( 'NONE', #45927, #18739 ) ;
#12899=EDGE_CURVE ( 'NONE', #9878, #11697, #37357, .T. ) ;
#12918=LINE ( 'NONE', #27313, #16937 ) ;
#12930=ORIENTED_EDGE ( 'NONE', *, *, #12430, .F. ) ;
#12966=DIRECTION ( 'NONE',  ( 1.000000000000000000, 0.000000000000000000, 0.000000000000000000 ) ) ;
#12971=CARTESIAN_POINT ( 'NONE',  ( 0.1733357866104492107, 0.3740157480314960647, 1.025733466389925352 ) ) ;
#12984=ORIENTED_EDGE ( 'NONE', *, *, #21541, .F. ) ;
#13047=LINE ( 'NONE', #6464, #20243 ) ;
#13066=CIRCLE ( 'NONE', #35986, 0.7874015748031496509 ) ;
#13085=EDGE_CURVE ( 'NONE', #42441, #17962, #41191, .T. ) ;
#13101=CIRCLE ( 'NONE', #23786, 0.1574803149606300579 ) ;
#13116=EDGE_CURVE ( 'NONE', #8447, #30501, #1843, .T. ) ;
#13139=DIRECTION ( 'NONE',  ( 0.8191520442889893561, -0.4519843998600455715, 0.3531289150159241386 ) ) ;
#13166=DIRECTION ( 'NONE',  ( 0.000000000000000000, -0.7880107536067206819, 0.6156614753256598460 ) ) ;
#13170=VECTOR ( 'NONE', #44642, 39.37007874015748143 ) ;
#13225=ORIENTED_EDGE ( 'NONE', *, *, #12430, .T. ) ;
#13302=PLANE ( 'NONE',  #18027 ) ;
#13342=DIRECTION ( 'NONE',  ( -1.000000000000000000, 0.000000000000000000, 0.000000000000000000 ) ) ;
#13406=EDGE_LOOP ( 'NONE', ( #37037, #11576, #21512, #20266 ) ) ;
#13453=ORIENTED_EDGE ( 'NONE', *, *, #11118, .T. ) ;
#13571=ORIENTED_EDGE ( 'NONE', *, *, #17755, .T. ) ;
#13623=ORIENTED_EDGE ( 'NONE', *, *, #20913, .F. ) ;
#13679=VERTEX_POINT ( 'NONE', #23384 ) ;
#13686=EDGE_CURVE ( 'NONE', #9939, #42894, #30132, .T. ) ;
#13754=DIRECTION ( 'NONE',  ( 1.000000000000000000, 0.000000000000000000, 0.000000000000000000 ) ) ;
#13761=DIRECTION ( 'NONE',  ( 6.944548107256202097E-15, 0.7880107536067212370, -0.6156614753256591799 ) ) ;
#13790=ORIENTED_EDGE ( 'NONE', *, *, #8708, .T. ) ;
#13793=CARTESIAN_POINT ( 'NONE',  ( 0.000000000000000000, 0.1473293504822035527, -0.9532488779249704836 ) ) ;
#13824=LINE ( 'NONE', #42783, #19226 ) ;
#13966=CYLINDRICAL_SURFACE ( 'NONE', #16773, 0.1864803149606298893 ) ;
#14003=CIRCLE ( 'NONE', #10179, 0.02899999999999988351 ) ;
#14041=CARTESIAN_POINT ( 'NONE',  ( 0.2759478392031617933, 0.3740157480314960647, 1.713085361781125915 ) ) ;
#14065=ORIENTED_EDGE ( 'NONE', *, *, #31827, .F. ) ;
#14079=EDGE_CURVE ( 'NONE', #15113, #30501, #18315, .T. ) ;
#14134=AXIS2_PLACEMENT_3D ( 'NONE', #15495, #30139, #44679 ) ;
#14145=DIRECTION ( 'NONE',  ( -1.000000000000000000, 0.000000000000000000, 0.000000000000000000 ) ) ;
#14156=LINE ( 'NONE', #24939, #4527 ) ;
#14174=VECTOR ( 'NONE', #40434, 39.37007874015748143 ) ;
#14248=ORIENTED_EDGE ( 'NONE', *, *, #27109, .T. ) ;
#14254=ADVANCED_FACE ( 'NONE', ( #43926 ), #36978, .T. ) ;
#14364=EDGE_CURVE ( 'NONE', #13679, #1767, #6792, .T. ) ;
#14432=DIRECTION ( 'NONE',  ( 1.000000000000000000, 0.000000000000000000, -7.083454193571960199E-15 ) ) ;
#14444=DIRECTION ( 'NONE',  ( 0.000000000000000000, 0.1045284632676499598, -0.9945218953682736229 ) ) ;
#14475=DIRECTION ( 'NONE',  ( -5.159318851433039196E-16, -0.6156614753256610673, -0.7880107536067199048 ) ) ;
#14520=EDGE_CURVE ( 'NONE', #34914, #2197, #3005, .T. ) ;
#14533=ADVANCED_FACE ( 'NONE', ( #5082 ), #15423, .T. ) ;
#14614=CARTESIAN_POINT ( 'NONE',  ( 0.000000000000000000, 0.3740157480314960647, 0.9783464566929134243 ) ) ;
#14659=CARTESIAN_POINT ( 'NONE',  ( 0.4736248074375464800, 1.798092712879862276, -3.826876940038421715 ) ) ;
#14671=FACE_OUTER_BOUND ( 'NONE', #39654, .T. ) ;
#14715=CARTESIAN_POINT ( 'NONE',  ( 0.1574803149606299191, 1.086379535891623949, -0.03715491745706121784 ) ) ;
#14731=DIRECTION ( 'NONE',  ( 1.000000000000000000, 2.114720919224289611E-16, 0.000000000000000000 ) ) ;
#14759=CARTESIAN_POINT ( 'NONE',  ( 0.4736248074375433714, 2.559880088878740079, -3.648497683167389649 ) ) ;
#14787=CIRCLE ( 'NONE', #26292, 0.1574803149606300579 ) ;
#14954=EDGE_LOOP ( 'NONE', ( #16872, #9471, #6621, #15891 ) ) ;
#14969=VECTOR ( 'NONE', #38807, 39.37007874015748143 ) ;
#14973=CARTESIAN_POINT ( 'NONE',  ( 0.2362204724409449064, 0.3740157480314960647, 0.9783464566929134243 ) ) ;
#15032=CIRCLE ( 'NONE', #34163, 0.7874015748031496509 ) ;
#15053=FACE_OUTER_BOUND ( 'NONE', #2944, .T. ) ;
#15111=ORIENTED_EDGE ( 'NONE', *, *, #44348, .T. ) ;
#15113=VERTEX_POINT ( 'NONE', #15654 ) ;
#15156=LINE ( 'NONE', #44346, #12494 ) ;
#15201=CARTESIAN_POINT ( 'NONE',  ( 0.1184675242425320824, 0.3740157480314960647, 1.713085361781127913 ) ) ;
#15203=AXIS2_PLACEMENT_3D ( 'NONE', #7824, #148, #33743 ) ;
#15226=ORIENTED_EDGE ( 'NONE', *, *, #22130, .T. ) ;
#15270=CARTESIAN_POINT ( 'NONE',  ( 0.2759478392031617933, -0.09842519685039370636, 1.713085361781125915 ) ) ;
#15329=DIRECTION ( 'NONE',  ( 5.310452730157438139E-15, 0.7880107536067220142, -0.6156614753256581807 ) ) ;
#15349=CARTESIAN_POINT ( 'NONE',  ( 0.2759478392031617933, -0.5708661417322835607, 1.713085361781125915 ) ) ;
#15386=DIRECTION ( 'NONE',  ( 0.000000000000000000, 0.000000000000000000, 1.000000000000000000 ) ) ;
#15423=CYLINDRICAL_SURFACE ( 'NONE', #35163, 0.7874015748031496509 ) ;
#15478=DIRECTION ( 'NONE',  ( -9.917966281713120965E-31, 1.000000000000000000, -1.406820448837680035E-16 ) ) ;
#15493=ORIENTED_EDGE ( 'NONE', *, *, #38625, .T. ) ;
#15495=CARTESIAN_POINT ( 'NONE',  ( 0.2362204724409449064, 0.3740157480314960647, 0.9783464566929134243 ) ) ;
#15518=ORIENTED_EDGE ( 'NONE', *, *, #16733, .T. ) ;
#15553=CARTESIAN_POINT ( 'NONE',  ( 0.1574803149606299191, 0.6241017553149685870, 0.3240160679609074834 ) ) ;
#15572=ORIENTED_EDGE ( 'NONE', *, *, #18368, .F. ) ;
#15636=ADVANCED_FACE ( 'NONE', ( #23009 ), #33823, .T. ) ;
#15654=CARTESIAN_POINT ( 'NONE',  ( 0.2383973256948909436, -0.5708661417322835607, 1.112073044918588494 ) ) ;
#15707=DIRECTION ( 'NONE',  ( -0.8191520442889947962, 0.4519843998600418522, -0.3531289150159164225 ) ) ;
#15717=CARTESIAN_POINT ( 'NONE',  ( 0.4399002236966062518, 0.8539303365987028771, -1.004656681308842447 ) ) ;
#15768=EDGE_CURVE ( 'NONE', #38536, #4180, #32950, .T. ) ;
#15791=VECTOR ( 'NONE', #45190, 39.37007874015748143 ) ;
#15822=DIRECTION ( 'NONE',  ( -1.000000000000000000, 5.464378949326940770E-15, -4.275490733183370330E-15 ) ) ;
#15852=CARTESIAN_POINT ( 'NONE',  ( -2.048885995248196921E-16, 1.086379535891622172, -0.03715491745705894189 ) ) ;
#15873=ADVANCED_FACE ( 'NONE', ( #38805 ), #2137, .F. ) ;
#15891=ORIENTED_EDGE ( 'NONE', *, *, #44348, .F. ) ;
#15905=CARTESIAN_POINT ( 'NONE',  ( 0.4736248074375866701, -0.09842519685039370636, 1.713085361781129690 ) ) ;
#15918=DIRECTION ( 'NONE',  ( 1.000000000000000000, 2.114720919224289611E-16, 0.000000000000000000 ) ) ;
#15941=LINE ( 'NONE', #801, #28394 ) ;
#15942=ORIENTED_EDGE ( 'NONE', *, *, #30758, .T. ) ;
#16005=VECTOR ( 'NONE', #16451, 39.37007874015748143 ) ;
#16044=DIRECTION ( 'NONE',  ( -0.000000000000000000, 1.000000000000000000, 0.000000000000000000 ) ) ;
#16069=PLANE ( 'NONE',  #4948 ) ;
#16086=AXIS2_PLACEMENT_3D ( 'NONE', #23598, #38211, #27465 ) ;
#16125=ORIENTED_EDGE ( 'NONE', *, *, #18830, .F. ) ;
#16132=VECTOR ( 'NONE', #20973, 39.37007874015748854 ) ;
#16188=CARTESIAN_POINT ( 'NONE',  ( 0.1184675242425352465, -0.09842519685039370636, 2.185526306663015728 ) ) ;
#16199=ORIENTED_EDGE ( 'NONE', *, *, #22462, .F. ) ;
#16302=CARTESIAN_POINT ( 'NONE',  ( 0.4736248074375449257, 2.177585298233984279, -3.731703755406948986 ) ) ;
#16346=EDGE_LOOP ( 'NONE', ( #1404, #24613, #27905, #25913 ) ) ;
#16382=PRODUCT_CONTEXT ( 'NONE', #41312, 'mechanical' ) ;
#16421=LINE ( 'NONE', #45616, #42810 ) ;
#16427=EDGE_CURVE ( 'NONE', #183, #7776, #9283, .T. ) ;
#16451=DIRECTION ( 'NONE',  ( -1.000000000000000000, -5.372880794957870593E-15, 4.197754538034584604E-15 ) ) ;
#16561=EDGE_CURVE ( 'NONE', #35279, #21057, #13101, .T. ) ;
#16570=EDGE_CURVE ( 'NONE', #17791, #36844, #1542, .T. ) ;
#16582=LINE ( 'NONE', #38373, #35415 ) ;
#16597=ORIENTED_EDGE ( 'NONE', *, *, #16561, .F. ) ;
#16646=ADVANCED_FACE ( 'NONE', ( #5378 ), #19527, .T. ) ;
#16733=EDGE_CURVE ( 'NONE', #39408, #32565, #36796, .T. ) ;
#16734=LINE ( 'NONE', #27794, #9333 ) ;
#16753=AXIS2_PLACEMENT_3D ( 'NONE', #22710, #32818, #43803 ) ;
#16773=AXIS2_PLACEMENT_3D ( 'NONE', #35777, #31487, #34852 ) ;
#16780=ADVANCED_FACE ( 'NONE', ( #17349 ), #36039, .F. ) ;
#16832=EDGE_CURVE ( 'NONE', #19538, #45189, #15941, .T. ) ;
#16863=DIRECTION ( 'NONE',  ( -5.464378949326941559E-15, -1.000000000000000000, 0.000000000000000000 ) ) ;
#16872=ORIENTED_EDGE ( 'NONE', *, *, #39267, .F. ) ;
#16876=AXIS2_PLACEMENT_3D ( 'NONE', #39376, #2255, #31982 ) ;
#16879=CARTESIAN_POINT ( 'NONE',  ( 0.1574803149606299191, 3.616083068348484413E-17, -0.2952755905511810774 ) ) ;
#16937=VECTOR ( 'NONE', #5465, 39.37007874015748143 ) ;
#16973=CARTESIAN_POINT ( 'NONE',  ( 0.2383973256948878072, 0.3740157480314960647, 1.112073044918586717 ) ) ;
#16990=ORIENTED_EDGE ( 'NONE', *, *, #24562, .F. ) ;
#16998=DIRECTION ( 'NONE',  ( 0.000000000000000000, 0.000000000000000000, -1.000000000000000000 ) ) ;
#17010=VECTOR ( 'NONE', #31845, 39.37007874015748854 ) ;
#17073=LINE ( 'NONE', #12798, #1671 ) ;
#17090=LINE ( 'NONE', #2700, #38462 ) ;
#17118=ORIENTED_EDGE ( 'NONE', *, *, #2162, .T. ) ;
#17174=AXIS2_PLACEMENT_3D ( 'NONE', #25330, #39918, #3515 ) ;
#17239=DIRECTION ( 'NONE',  ( 0.5735764363510417185, 0.6455006197386566891, -0.5043203561029927506 ) ) ;
#17263=AXIS2_PLACEMENT_3D ( 'NONE', #37794, #26316, #11691 ) ;
#17295=CARTESIAN_POINT ( 'NONE',  ( 0.1574803149606299191, 0.4666052258408008302, -0.7025346432751023995 ) ) ;
#17349=FACE_OUTER_BOUND ( 'NONE', #41906, .T. ) ;
#17350=DIRECTION ( 'NONE',  ( 2.943801717310645197E-16, -1.000000000000000000, -2.197428715927220134E-15 ) ) ;
#17377=EDGE_LOOP ( 'NONE', ( #15518, #29698, #27038, #22237 ) ) ;
#17432=FACE_OUTER_BOUND ( 'NONE', #19328, .T. ) ;
#17479=DIRECTION ( 'NONE',  ( 0.000000000000000000, 0.000000000000000000, -1.000000000000000000 ) ) ;
#17527=ADVANCED_FACE ( 'NONE', ( #1698 ), #30969, .T. ) ;
#17533=CARTESIAN_POINT ( 'NONE',  ( 0.4736248074375464800, 1.798092712879862276, -3.826876940038421715 ) ) ;
#17547=FACE_OUTER_BOUND ( 'NONE', #3851, .T. ) ;
#17550=CARTESIAN_POINT ( 'NONE',  ( 0.000000000000000000, 0.000000000000000000, 0.2952755905511810774 ) ) ;
#17618=LINE ( 'NONE', #39642, #36035 ) ;
#17737=DIRECTION ( 'NONE',  ( -1.000000000000000000, 0.000000000000000000, 0.000000000000000000 ) ) ;
#17754=VECTOR ( 'NONE', #2806, 39.37007874015748854 ) ;
#17755=EDGE_CURVE ( 'NONE', #31929, #2197, #45291, .T. ) ;
#17791=VERTEX_POINT ( 'NONE', #12971 ) ;
#17792=VECTOR ( 'NONE', #31728, 39.37007874015748854 ) ;
#17805=EDGE_CURVE ( 'NONE', #13679, #44149, #43585, .T. ) ;
#17812=DIRECTION ( 'NONE',  ( 1.831190596606011519E-15, -0.7880107536067199048, 0.6156614753256609562 ) ) ;
#17947=CARTESIAN_POINT ( 'NONE',  ( 0.1184675242425352465, 0.3740157480314960647, 2.185526306663015728 ) ) ;
#17962=VERTEX_POINT ( 'NONE', #25410 ) ;
#17974=EDGE_LOOP ( 'NONE', ( #20574, #25857, #12572, #41783 ) ) ;
#18020=VECTOR ( 'NONE', #19469, 39.37007874015748854 ) ;
#18027=AXIS2_PLACEMENT_3D ( 'NONE', #27231, #45862, #23383 ) ;
#18097=DIRECTION ( 'NONE',  ( 0.000000000000000000, -0.1045284632676499459, 0.9945218953682736229 ) ) ;
#18099=ORIENTED_EDGE ( 'NONE', *, *, #3053, .F. ) ;
#18107=LINE ( 'NONE', #14041, #42831 ) ;
#18153=CARTESIAN_POINT ( 'NONE',  ( 0.1574803149606299191, 0.1473293504822035527, -0.9532488779249704836 ) ) ;
#18180=DIRECTION ( 'NONE',  ( 0.6018150231520440485, 0.000000000000000000, 0.7986355100472960489 ) ) ;
#18181=LINE ( 'NONE', #36410, #14174 ) ;
#18193=PRESENTATION_STYLE_ASSIGNMENT (( #10788 ) ) ;
#18249=LINE ( 'NONE', #14659, #267 ) ;
#18315=CIRCLE ( 'NONE', #45074, 0.1864803149606299448 ) ;
#18317=DIRECTION ( 'NONE',  ( -1.000000000000000000, 0.000000000000000000, 7.155734338404321376E-15 ) ) ;
#18320=DIRECTION ( 'NONE',  ( -5.159318851433079625E-16, -0.6156614753256609562, -0.7880107536067197938 ) ) ;
#18331=LINE ( 'NONE', #29640, #23898 ) ;
#18361=VERTEX_POINT ( 'NONE', #46185 ) ;
#18368=EDGE_CURVE ( 'NONE', #34914, #36844, #16734, .T. ) ;
#18389=ORIENTED_EDGE ( 'NONE', *, *, #25778, .T. ) ;
#18411=CARTESIAN_POINT ( 'NONE',  ( 0.3161444924769519216, 1.488499961090669288, -0.3513258257898460579 ) ) ;
#18418=EDGE_LOOP ( 'NONE', ( #42036, #37758, #15493, #12984 ) ) ;
#18448=ADVANCED_FACE ( 'NONE', ( #41620, #8829 ), #45702, .F. ) ;
#18532=DIRECTION ( 'NONE',  ( 0.6018150231520440485, 0.000000000000000000, 0.7986355100472960489 ) ) ;
#18535=VECTOR ( 'NONE', #2164, 39.37007874015748143 ) ;
#18566=VERTEX_POINT ( 'NONE', #43298 ) ;
#18592=PLANE ( 'NONE',  #43709 ) ;
#18594=AXIS2_PLACEMENT_3D ( 'NONE', #14973, #3923, #15918 ) ;
#18618=CYLINDRICAL_SURFACE ( 'NONE', #17263, 0.2952755905511810774 ) ;
#18644=EDGE_LOOP ( 'NONE', ( #5673, #12930, #38691, #13790 ) ) ;
#18684=LINE ( 'NONE', #15349, #9817 ) ;
#18691=EDGE_LOOP ( 'NONE', ( #1867, #43742, #15572, #31815 ) ) ;
#18694=CARTESIAN_POINT ( 'NONE',  ( 0.3161444924769519216, 1.488499961090669288, -0.3513258257898460579 ) ) ;
#18707=DIRECTION ( 'NONE',  ( 1.000000000000000000, 5.372880794957870593E-15, -4.197754538034584604E-15 ) ) ;
#18721=LINE ( 'NONE', #39577, #45233 ) ;
#18725=CARTESIAN_POINT ( 'NONE',  ( 0.1574803149606299191, 0.3740157480314960647, 0.9783464566929134243 ) ) ;
#18734=VERTEX_POINT ( 'NONE', #44463 ) ;
#18739=VECTOR ( 'NONE', #13139, 39.37007874015748854 ) ;
#18765=DIRECTION ( 'NONE',  ( -5.244653365444468611E-15, 0.2126700594527759225, -0.9771240687918565371 ) ) ;
#18776=EDGE_CURVE ( 'NONE', #7776, #24150, #36109, .T. ) ;
#18784=DIRECTION ( 'NONE',  ( -7.047314121155773299E-15, 0.000000000000000000, 1.000000000000000000 ) ) ;
#18826=EDGE_CURVE ( 'NONE', #44566, #22983, #30760, .T. ) ;
#18830=EDGE_CURVE ( 'NONE', #30077, #7776, #34661, .T. ) ;
#18871=ORIENTED_EDGE ( 'NONE', *, *, #13116, .T. ) ;
#18877=EDGE_LOOP ( 'NONE', ( #44108, #15226, #23778, #11992 ) ) ;
#18891=DIRECTION ( 'NONE',  ( -5.464378949326941559E-15, -1.000000000000000000, 0.000000000000000000 ) ) ;
#18937=EDGE_LOOP ( 'NONE', ( #43498, #36237, #40183, #20675 ) ) ;
#18950=DIRECTION ( 'NONE',  ( -5.159318851433039196E-16, -0.6156614753256610673, -0.7880107536067199048 ) ) ;
#18996=CARTESIAN_POINT ( 'NONE',  ( 0.4736248074375882244, -0.09842519685039370636, 1.555605046820500048 ) ) ;
#19014=CARTESIAN_POINT ( 'NONE',  ( 0.1184675242425320824, -0.09842519685039370636, 1.713085361781127913 ) ) ;
#19015=DIRECTION ( 'NONE',  ( 2.943801717310650128E-16, -1.000000000000000000, -2.355041373848525230E-15 ) ) ;
#19026=ORIENTED_EDGE ( 'NONE', *, *, #24896, .F. ) ;
#19032=EDGE_CURVE ( 'NONE', #8850, #21023, #12392, .T. ) ;
#19071=CYLINDRICAL_SURFACE ( 'NONE', #15203, 0.2952755905511810774 ) ;
#19086=FACE_OUTER_BOUND ( 'NONE', #17974, .T. ) ;
#19129=EDGE_LOOP ( 'NONE', ( #11010, #9226, #28097, #19990 ) ) ;
#19137=CARTESIAN_POINT ( 'NONE',  ( 0.2871444924769520068, 1.495705267341507883, -0.3569552279982047271 ) ) ;
#19166=DIRECTION ( 'NONE',  ( 4.750595374550219683E-16, 0.6156614753256610673, 0.7880107536067199048 ) ) ;
#19173=DIRECTION ( 'NONE',  ( 1.000000000000000000, 0.000000000000000000, 0.000000000000000000 ) ) ;
#19195=ADVANCED_FACE ( 'NONE', ( #29154 ), #22378, .F. ) ;
#19204=EDGE_CURVE ( 'NONE', #22479, #19538, #29862, .T. ) ;
#19226=VECTOR ( 'NONE', #45930, 39.37007874015748854 ) ;
#19227=ORIENTED_EDGE ( 'NONE', *, *, #31671, .F. ) ;
#19262=PLANE ( 'NONE',  #22436 ) ;
#19325=DIRECTION ( 'NONE',  ( 0.000000000000000000, -1.000000000000000000, 0.000000000000000000 ) ) ;
#19328=EDGE_LOOP ( 'NONE', ( #38150, #37351, #12819, #30746 ) ) ;
#19333=CARTESIAN_POINT ( 'NONE',  ( 0.1864803149606299171, 1.086379535891623949, -0.03715491745706168969 ) ) ;
#19371=ORIENTED_EDGE ( 'NONE', *, *, #9854, .F. ) ;
#19379=CARTESIAN_POINT ( 'NONE',  ( 0.3161444924769519216, 1.495705267341507883, -0.3569552279982051712 ) ) ;
#19395=ORIENTED_EDGE ( 'NONE', *, *, #7535, .F. ) ;
#19416=EDGE_LOOP ( 'NONE', ( #40077, #36375, #25803, #32862 ) ) ;
#19417=ORIENTED_EDGE ( 'NONE', *, *, #20654, .T. ) ;
#19423=( CONVERSION_BASED_UNIT ( 'INCH', #40733 ) LENGTH_UNIT ( ) NAMED_UNIT ( #46381 ) ) ;
#19436=DIRECTION ( 'NONE',  ( 5.159318851433039196E-16, 0.6156614753256609562, 0.7880107536067197938 ) ) ;
#19469=DIRECTION ( 'NONE',  ( -6.944548107256197364E-15, -0.7880107536067206819, 0.6156614753256598460 ) ) ;
#19473=CARTESIAN_POINT ( 'NONE',  ( 0.000000000000000000, 0.1473293504822035527, -0.5595480905233944924 ) ) ;
#19527=PLANE ( 'NONE',  #42868 ) ;
#19538=VERTEX_POINT ( 'NONE', #34142 ) ;
#19574=DIRECTION ( 'NONE',  ( 2.710505431213762009E-17, 0.6156614753256599570, 0.7880107536067207930 ) ) ;
#19587=CARTESIAN_POINT ( 'NONE',  ( 0.3161444924769130083, 2.559880088878740079, -3.648497683167389649 ) ) ;
#19616=LINE ( 'NONE', #20089, #9281 ) ;
#19620=ORIENTED_EDGE ( 'NONE', *, *, #47295, .F. ) ;
#19656=EDGE_CURVE ( 'NONE', #6130, #35620, #28851, .T. ) ;
#19677=AXIS2_PLACEMENT_3D ( 'NONE', #21149, #42940, #4054 ) ;
#19684=CARTESIAN_POINT ( 'NONE',  ( 0.2362204724409449064, -0.5708661417322835607, 0.9783464566929134243 ) ) ;
#19704=DIRECTION ( 'NONE',  ( 5.377642775528101993E-15, -1.000000000000000000, 0.000000000000000000 ) ) ;
#19731=DIRECTION ( 'NONE',  ( 0.000000000000000000, -1.000000000000000000, 0.000000000000000000 ) ) ;
#19747=ORIENTED_EDGE ( 'NONE', *, *, #30758, .F. ) ;
#19756=EDGE_CURVE ( 'NONE', #42619, #28693, #32225, .T. ) ;
#19791=DIRECTION ( 'NONE',  ( 1.000000000000000000, -5.472378587457090550E-15, 4.280079833532960850E-15 ) ) ;
#19848=DIRECTION ( 'NONE',  ( 0.000000000000000000, 1.000000000000000000, 0.000000000000000000 ) ) ;
#19853=CARTESIAN_POINT ( 'NONE',  ( 0.1574803149606299191, 0.08719492171395729074, -0.5641677032617165022 ) ) ;
#19894=( NAMED_UNIT ( * ) PLANE_ANGLE_UNIT ( ) SI_UNIT ( $, .RADIAN. ) ) ;
#19990=ORIENTED_EDGE ( 'NONE', *, *, #19204, .F. ) ;
#20020=DIRECTION ( 'NONE',  ( -5.244653365444468611E-15, 0.2126700594527759225, -0.9771240687918565371 ) ) ;
#20032=CARTESIAN_POINT ( 'NONE',  ( 0.2871444924769515628, 0.9382165298418956301, -1.070508272602716637 ) ) ;
#20060=ORIENTED_EDGE ( 'NONE', *, *, #20654, .F. ) ;
#20089=CARTESIAN_POINT ( 'NONE',  ( 0.3161444924769145626, 1.890321945096787193, -4.194630839571732217 ) ) ;
#20090=DIRECTION ( 'NONE',  ( 2.710505431213758620E-17, -0.6156614753256599570, -0.7880107536067207930 ) ) ;
#20124=AXIS2_PLACEMENT_3D ( 'NONE', #2570, #20090, #13166 ) ;
#20136=CARTESIAN_POINT ( 'NONE',  ( 0.1574803149606299191, -5.122214988120488358E-16, -8.878505979408856939E-16 ) ) ;
#20243=VECTOR ( 'NONE', #8961, 39.37007874015748854 ) ;
#20260=DIRECTION ( 'NONE',  ( -3.580839449783114748E-16, 0.6156614753256610673, 0.7880107536067199048 ) ) ;
#20266=ORIENTED_EDGE ( 'NONE', *, *, #17805, .F. ) ;
#20324=CARTESIAN_POINT ( 'NONE',  ( 0.1184675242425320824, -0.5708661417322835607, 1.713085361781127913 ) ) ;
#20343=ORIENTED_EDGE ( 'NONE', *, *, #9816, .F. ) ;
#20407=EDGE_CURVE ( 'NONE', #9939, #36104, #28414, .T. ) ;
#20410=PRODUCT_DEFINITION ( 'UNKNOWN', '', #22435, #24535 ) ;
#20414=CYLINDRICAL_SURFACE ( 'NONE', #44793, 0.3937007874015748254 ) ;
#20429=AXIS2_PLACEMENT_3D ( 'NONE', #26685, #45328, #12545 ) ;
#20474=FACE_OUTER_BOUND ( 'NONE', #4445, .T. ) ;
#20501=AXIS2_PLACEMENT_3D ( 'NONE', #232, #40479, #6959 ) ;
#20509=EDGE_CURVE ( 'NONE', #43030, #6306, #17618, .T. ) ;
#20549=PLANE ( 'NONE',  #23852 ) ;
#20574=ORIENTED_EDGE ( 'NONE', *, *, #36269, .F. ) ;
#20583=DIRECTION ( 'NONE',  ( 7.659124183791938496E-17, -1.000000000000000000, 1.016400108624885935E-16 ) ) ;
#20635=FACE_BOUND ( 'NONE', #45464, .T. ) ;
#20652=CARTESIAN_POINT ( 'NONE',  ( -0.4955489724641236604, 0.3740157480314960647, 0.3997690233743834698 ) ) ;
#20654=EDGE_CURVE ( 'NONE', #28784, #24486, #7774, .T. ) ;
#20675=ORIENTED_EDGE ( 'NONE', *, *, #40562, .T. ) ;
#20684=EDGE_CURVE ( 'NONE', #8447, #27121, #26002, .T. ) ;
#20714=EDGE_CURVE ( 'NONE', #8512, #24150, #11631, .T. ) ;
#20746=ORIENTED_EDGE ( 'NONE', *, *, #1075, .F. ) ;
#20761=LINE ( 'NONE', #43029, #2683 ) ;
#20781=DIRECTION ( 'NONE',  ( -1.000000000000000000, -5.372880794957750686E-15, 4.197754538034109710E-15 ) ) ;
#20824=CARTESIAN_POINT ( 'NONE',  ( 0.000000000000000000, 0.3883517482604913473, -0.6419475548153091848 ) ) ;
#20826=EDGE_CURVE ( 'NONE', #24150, #17791, #38740, .T. ) ;
#20830=VECTOR ( 'NONE', #18532, 39.37007874015748854 ) ;
#20860=AXIS2_PLACEMENT_3D ( 'NONE', #25692, #32652, #10835 ) ;
#20876=DIRECTION ( 'NONE',  ( 0.000000000000000000, -2.355041373848501170E-15, 1.000000000000000000 ) ) ;
#20894=VECTOR ( 'NONE', #39276, 39.37007874015748143 ) ;
#20897=PLANE ( 'NONE',  #33382 ) ;
#20913=EDGE_CURVE ( 'NONE', #40723, #7704, #45434, .T. ) ;
#20940=ORIENTED_EDGE ( 'NONE', *, *, #35921, .T. ) ;
#20973=DIRECTION ( 'NONE',  ( 0.000000000000000000, -0.1045284632676499459, 0.9945218953682736229 ) ) ;
#20991=DIRECTION ( 'NONE',  ( 0.000000000000000000, 1.000000000000000000, 6.980778575359379259E-17 ) ) ;
#20999=ORIENTED_EDGE ( 'NONE', *, *, #35855, .T. ) ;
#21016=DIRECTION ( 'NONE',  ( 0.000000000000000000, 0.000000000000000000, 1.000000000000000000 ) ) ;
#21023=VERTEX_POINT ( 'NONE', #14759 ) ;
#21039=EDGE_LOOP ( 'NONE', ( #36117, #29659, #21538, #37654 ) ) ;
#21055=AXIS2_PLACEMENT_3D ( 'NONE', #34265, #15822, #5237 ) ;
#21057=VERTEX_POINT ( 'NONE', #6835 ) ;
#21149=CARTESIAN_POINT ( 'NONE',  ( 0.1184675242425320824, -0.09842519685039370636, 1.713085361781127913 ) ) ;
#21175=ORIENTED_EDGE ( 'NONE', *, *, #44030, .T. ) ;
#21248=ORIENTED_EDGE ( 'NONE', *, *, #19756, .F. ) ;
#21388=CARTESIAN_POINT ( 'NONE',  ( 0.3161444924769554743, 1.357244529069700612, -1.397888825503271759 ) ) ;
#21512=ORIENTED_EDGE ( 'NONE', *, *, #44949, .T. ) ;
#21530=EDGE_CURVE ( 'NONE', #40723, #13679, #45241, .T. ) ;
#21538=ORIENTED_EDGE ( 'NONE', *, *, #22025, .T. ) ;
#21541=EDGE_CURVE ( 'NONE', #5864, #43030, #46899, .T. ) ;
#21551=AXIS2_PLACEMENT_3D ( 'NONE', #11213, #19325, #29924 ) ;
#21556=AXIS2_PLACEMENT_3D ( 'NONE', #7819, #29458, #44003 ) ;
#21559=FACE_OUTER_BOUND ( 'NONE', #25663, .T. ) ;
#21661=ORIENTED_EDGE ( 'NONE', *, *, #36047, .F. ) ;
#21680=DIRECTION ( 'NONE',  ( -9.420165495393842173E-15, -0.7880107536067199048, 0.6156614753256609562 ) ) ;
#21710=AXIS2_PLACEMENT_3D ( 'NONE', #31704, #35299, #46289 ) ;
#21712=ORIENTED_EDGE ( 'NONE', *, *, #4543, .T. ) ;
#21719=ADVANCED_FACE ( 'NONE', ( #44469 ), #34207, .F. ) ;
#21728=ORIENTED_EDGE ( 'NONE', *, *, #7535, .T. ) ;
#21732=ORIENTED_EDGE ( 'NONE', *, *, #35921, .F. ) ;
#21793=( CONVERSION_BASED_UNIT ( 'INCH', #7168 ) LENGTH_UNIT ( ) NAMED_UNIT ( #33833 ) ) ;
#21807=DIRECTION ( 'NONE',  ( 0.000000000000000000, -0.6156614753256599570, -0.7880107536067207930 ) ) ;
#21870=ORIENTED_EDGE ( 'NONE', *, *, #44289, .F. ) ;
#21995=EDGE_LOOP ( 'NONE', ( #2127, #710, #36847, #18871 ) ) ;
#22006=DIRECTION ( 'NONE',  ( 6.944548107256202097E-15, 0.7880107536067212370, -0.6156614753256591799 ) ) ;
#22017=FILL_AREA_STYLE ('',( #432 ) ) ;
#22025=EDGE_CURVE ( 'NONE', #9878, #22983, #18331, .T. ) ;
#22075=CARTESIAN_POINT ( 'NONE',  ( 0.4736248074375818407, 0.9382165298418937427, -1.070508272602714639 ) ) ;
#22130=EDGE_CURVE ( 'NONE', #29781, #2057, #40344, .T. ) ;
#22148=LINE ( 'NONE', #563, #44431 ) ;
#22152=CARTESIAN_POINT ( 'NONE',  ( 0.1574803149606299191, -0.5708661417322835607, 0.9783464566929134243 ) ) ;
#22167=EDGE_LOOP ( 'NONE', ( #2588, #26151, #42026, #46031 ) ) ;
#22201=VECTOR ( 'NONE', #41591, 39.37007874015748143 ) ;
#22211=CARTESIAN_POINT ( 'NONE',  ( 0.1574803149606299191, -0.5708661417322835607, -6.991093932140394160E-17 ) ) ;
#22237=ORIENTED_EDGE ( 'NONE', *, *, #7951, .T. ) ;
#22257=VECTOR ( 'NONE', #19791, 39.37007874015748143 ) ;
#22378=PLANE ( 'NONE',  #46802 ) ;
#22379=DIRECTION ( 'NONE',  ( -2.891205793294680298E-16, 1.000000000000000000, 0.000000000000000000 ) ) ;
#22405=CARTESIAN_POINT ( 'NONE',  ( 0.2759478392031653460, 0.3740157480314960647, 2.185526306663015728 ) ) ;
#22435=PRODUCT_DEFINITION_FORMATION_WITH_SPECIFIED_SOURCE ( 'ANY', '', #29172, .NOT_KNOWN. ) ;
#22436=AXIS2_PLACEMENT_3D ( 'NONE', #33916, #40573, #36544 ) ;
#22462=EDGE_CURVE ( 'NONE', #34892, #42619, #17090, .T. ) ;
#22479=VERTEX_POINT ( 'NONE', #24296 ) ;
#22481=ORIENTED_EDGE ( 'NONE', *, *, #3021, .F. ) ;
#22493=EDGE_CURVE ( 'NONE', #6130, #9939, #39352, .T. ) ;
#22506=CARTESIAN_POINT ( 'NONE',  ( 0.4736248074375818407, 1.101950626536848388, -0.8609381856333149230 ) ) ;
#22507=CARTESIAN_POINT ( 'NONE',  ( 0.1574803149606299191, 0.6241017553149685870, 0.3240160679609074834 ) ) ;
#22580=CARTESIAN_POINT ( 'NONE',  ( 0.1184675242425088648, -0.09842519685039370636, 1.555605046820498050 ) ) ;
#22624=DIRECTION ( 'NONE',  ( 1.885568995626964040E-16, 0.6156614753256598460, 0.7880107536067206819 ) ) ;
#22626=CARTESIAN_POINT ( 'NONE',  ( 0.2362204724409449064, 0.3740157480314960647, 0.9783464566929134243 ) ) ;
#22628=CARTESIAN_POINT ( 'NONE',  ( 0.1574803149606299191, 0.4668427075568346574, -0.7022306805398661478 ) ) ;
#22664=ORIENTED_EDGE ( 'NONE', *, *, #31147, .F. ) ;
#22693=DIRECTION ( 'NONE',  ( 1.000000000000000000, -4.402590611634445055E-17, 0.000000000000000000 ) ) ;
#22710=CARTESIAN_POINT ( 'NONE',  ( 0.1574803149606299191, 0.9876813667277579700, 0.7893767492247204531 ) ) ;
#22719=EDGE_CURVE ( 'NONE', #43976, #40723, #25449, .T. ) ;
#22732=CARTESIAN_POINT ( 'NONE',  ( 0.4736248074375818407, 0.4457451269443653552, -1.671447902550338815 ) ) ;
#22765=CARTESIAN_POINT ( 'NONE',  ( 0.000000000000000000, 0.9876813667277579700, 0.7893767492247204531 ) ) ;
#22783=AXIS2_PLACEMENT_3D ( 'NONE', #22626, #22379, #333 ) ;
#22939=ORIENTED_EDGE ( 'NONE', *, *, #34652, .F. ) ;
#22983=VERTEX_POINT ( 'NONE', #17550 ) ;
#22987=ORIENTED_EDGE ( 'NONE', *, *, #8556, .F. ) ;
#23009=FACE_OUTER_BOUND ( 'NONE', #41775, .T. ) ;
#23030=VECTOR ( 'NONE', #33925, 39.37007874015748143 ) ;
#23035=PLANE ( 'NONE',  #24405 ) ;
#23107=CARTESIAN_POINT ( 'NONE',  ( 0.1574803149606299191, -0.5708661417322835607, 0.9783464566929134243 ) ) ;
#23135=CARTESIAN_POINT ( 'NONE',  ( 0.04756641494945763188, 0.3740157480314960647, 1.120507485783946766 ) ) ;
#23137=LINE ( 'NONE', #16879, #31832 ) ;
#23266=ORIENTED_EDGE ( 'NONE', *, *, #12899, .F. ) ;
#23296=DIRECTION ( 'NONE',  ( -0.7986355100472959379, -2.891205793294678326E-16, 0.6018150231520442706 ) ) ;
#23313=EDGE_CURVE ( 'NONE', #8746, #15113, #15156, .T. ) ;
#23381=DIRECTION ( 'NONE',  ( -7.047314121155773299E-15, 0.000000000000000000, 1.000000000000000000 ) ) ;
#23383=DIRECTION ( 'NONE',  ( 1.000000000000000000, 4.379520288671465147E-30, 0.000000000000000000 ) ) ;
#23384=CARTESIAN_POINT ( 'NONE',  ( 0.1574803149606299191, 0.3883517482604913473, -0.6419475548153091848 ) ) ;
#23402=DIRECTION ( 'NONE',  ( 1.000000000000000000, 0.000000000000000000, -7.044195017643630340E-15 ) ) ;
#23444=ADVANCED_FACE ( 'NONE', ( #46426 ), #23469, .F. ) ;
#23469=PLANE ( 'NONE',  #20124 ) ;
#23549=EDGE_CURVE ( 'NONE', #33555, #44909, #11149, .T. ) ;
#23551=EDGE_LOOP ( 'NONE', ( #2537, #21712, #31556, #42722, #32974 ) ) ;
#23560=CARTESIAN_POINT ( 'NONE',  ( 0.4399002236966070845, 1.411419074098315019, -0.2911036367043311479 ) ) ;
#23575=LINE ( 'NONE', #24058, #40382 ) ;
#23598=CARTESIAN_POINT ( 'NONE',  ( 0.2871444924769520068, 1.495705267341507883, -0.3569552279982047271 ) ) ;
#23608=DIRECTION ( 'NONE',  ( 1.000000000000000000, -5.472378587457090550E-15, 4.280079833532960850E-15 ) ) ;
#23644=EDGE_CURVE ( 'NONE', #8746, #8447, #14003, .T. ) ;
#23702=ORIENTED_EDGE ( 'NONE', *, *, #2162, .F. ) ;
#23717=CARTESIAN_POINT ( 'NONE',  ( 0.4736248074375440931, 1.890321945096787193, -4.194630839571732217 ) ) ;
#23738=DIRECTION ( 'NONE',  ( 7.047314121155781188E-15, 0.000000000000000000, 1.000000000000000000 ) ) ;
#23757=EDGE_CURVE ( 'NONE', #24486, #2197, #31489, .T. ) ;
#23770=ORIENTED_EDGE ( 'NONE', *, *, #24615, .F. ) ;
#23778=ORIENTED_EDGE ( 'NONE', *, *, #4543, .F. ) ;
#23786=AXIS2_PLACEMENT_3D ( 'NONE', #5144, #30585, #23381 ) ;
#23829=DIRECTION ( 'NONE',  ( 1.000000000000000000, -5.464378949326940770E-15, 4.275490733183370330E-15 ) ) ;
#23834=ORIENTED_EDGE ( 'NONE', *, *, #22719, .T. ) ;
#23842=DIRECTION ( 'NONE',  ( -0.7986355100472960489, 0.000000000000000000, 0.6018150231520440485 ) ) ;
#23852=AXIS2_PLACEMENT_3D ( 'NONE', #45226, #31132, #41863 ) ;
#23898=VECTOR ( 'NONE', #37011, 39.37007874015748143 ) ;
#23903=CARTESIAN_POINT ( 'NONE',  ( 0.1184675242425285574, -0.5708661417322835607, 1.224299699984021661 ) ) ;
#23961=FACE_OUTER_BOUND ( 'NONE', #37989, .T. ) ;
#24026=DIRECTION ( 'NONE',  ( 0.000000000000000000, 0.000000000000000000, 1.000000000000000000 ) ) ;
#24058=CARTESIAN_POINT ( 'NONE',  ( 0.1733357866104492107, 0.3740157480314960647, 1.025733466389925352 ) ) ;
#24111=CARTESIAN_POINT ( 'NONE',  ( 0.1184675242425285574, 0.3740157480314960647, 1.224299699984021661 ) ) ;
#24150=VERTEX_POINT ( 'NONE', #41449 ) ;
#24156=DIRECTION ( 'NONE',  ( -5.411399086424348811E-15, -1.000000000000000000, 0.000000000000000000 ) ) ;
#24171=FACE_OUTER_BOUND ( 'NONE', #11184, .T. ) ;
#24172=CARTESIAN_POINT ( 'NONE',  ( 0.2759478392031499694, 0.000000000000000000, -1.945618984458255724E-15 ) ) ;
#24180=DIRECTION ( 'NONE',  ( -0.5735764363510409414, -0.6455006197386570221, 0.5043203561029929727 ) ) ;
#24195=ORIENTED_EDGE ( 'NONE', *, *, #13686, .T. ) ;
#24196=DIRECTION ( 'NONE',  ( -1.000000000000000000, 0.000000000000000000, 0.000000000000000000 ) ) ;
#24224=LINE ( 'NONE', #17947, #20894 ) ;
#24258=PLANE ( 'NONE',  #34818 ) ;
#24261=EDGE_LOOP ( 'NONE', ( #150, #46970, #688, #37729 ) ) ;
#24277=CIRCLE ( 'NONE', #25824, 0.2952755905511810774 ) ;
#24296=CARTESIAN_POINT ( 'NONE',  ( 0.1627249056762484491, 0.5419983459879520460, -0.7609487005970335671 ) ) ;
#24345=PLANE ( 'NONE',  #36030 ) ;
#24385=VERTEX_POINT ( 'NONE', #19587 ) ;
#24405=AXIS2_PLACEMENT_3D ( 'NONE', #1870, #2566, #37650 ) ;
#24434=ORIENTED_EDGE ( 'NONE', *, *, #20509, .F. ) ;
#24486=VERTEX_POINT ( 'NONE', #33210 ) ;
#24535=PRODUCT_DEFINITION_CONTEXT ( 'detailed design', #3971, 'design' ) ;
#24562=EDGE_CURVE ( 'NONE', #33555, #1767, #8237, .T. ) ;
#24579=VECTOR ( 'NONE', #39004, 39.37007874015748143 ) ;
#24604=FACE_OUTER_BOUND ( 'NONE', #9830, .T. ) ;
#24613=ORIENTED_EDGE ( 'NONE', *, *, #23644, .F. ) ;
#24615=EDGE_CURVE ( 'NONE', #2057, #43422, #5625, .T. ) ;
#24617=ADVANCED_FACE ( 'NONE', ( #25993 ), #19262, .F. ) ;
#24631=CARTESIAN_POINT ( 'NONE',  ( 0.4736248074375590811, 1.209494567139730359, -1.479906699140348447 ) ) ;
#24640=VECTOR ( 'NONE', #18765, 39.37007874015748143 ) ;
#24666=CARTESIAN_POINT ( 'NONE',  ( 0.4736248074375574713, 1.975221432870720495, -0.9622519263226653186 ) ) ;
#24673=AXIS2_PLACEMENT_3D ( 'NONE', #26928, #12066, #8446 ) ;
#24684=EDGE_CURVE ( 'NONE', #36924, #43976, #974, .T. ) ;
#24696=ORIENTED_EDGE ( 'NONE', *, *, #37545, .T. ) ;
#24721=FACE_OUTER_BOUND ( 'NONE', #19129, .T. ) ;
#24849=ORIENTED_EDGE ( 'NONE', *, *, #22493, .F. ) ;
#24865=CARTESIAN_POINT ( 'NONE',  ( 0.2871444924769515628, 0.9382165298418956301, -1.070508272602716637 ) ) ;
#24887=ORIENTED_EDGE ( 'NONE', *, *, #22493, .T. ) ;
#24896=EDGE_CURVE ( 'NONE', #43422, #30077, #24224, .T. ) ;
#24906=EDGE_CURVE ( 'NONE', #2197, #39408, #31656, .T. ) ;
#24931=ORIENTED_EDGE ( 'NONE', *, *, #35715, .F. ) ;
#24939=CARTESIAN_POINT ( 'NONE',  ( 0.1574803149606299191, 0.4003652867858621955, 0.7276473417831970103 ) ) ;
#24941=EDGE_LOOP ( 'NONE', ( #20060, #43411, #10396, #31603 ) ) ;
#24997=ORIENTED_EDGE ( 'NONE', *, *, #38625, .F. ) ;
#25023=CYLINDRICAL_SURFACE ( 'NONE', #6567, 0.5905511811023621549 ) ;
#25056=ORIENTED_EDGE ( 'NONE', *, *, #2146, .F. ) ;
#25072=CARTESIAN_POINT ( 'NONE',  ( 0.3161444924769527542, 1.025704337919492115, -1.138861239548320858 ) ) ;
#25099=FACE_OUTER_BOUND ( 'NONE', #17377, .T. ) ;
#25120=EDGE_LOOP ( 'NONE', ( #9593, #43569, #31733, #3135 ) ) ;
#25173=CARTESIAN_POINT ( 'NONE',  ( 0.2759478392031582961, -0.5708661417322835607, 1.214596435718460654 ) ) ;
#25249=EDGE_LOOP ( 'NONE', ( #26691, #13453, #30709, #39895 ) ) ;
#25291=AXIS2_PLACEMENT_3D ( 'NONE', #19684, #34327, #23296 ) ;
#25330=CARTESIAN_POINT ( 'NONE',  ( 0.08946752424252854552, 0.3740157480314960647, 1.224299699984021661 ) ) ;
#25356=DIRECTION ( 'NONE',  ( 1.000000000000000000, -4.710082747697002339E-15, 4.710082747697002339E-15 ) ) ;
#25410=CARTESIAN_POINT ( 'NONE',  ( 0.1574803149606299191, 0.4003652867858621955, 0.7276473417831970103 ) ) ;
#25449=CIRCLE ( 'NONE', #28527, 0.3937007874015747699 ) ;
#25489=DIRECTION ( 'NONE',  ( 0.000000000000000000, 0.000000000000000000, -1.000000000000000000 ) ) ;
#25520=ADVANCED_FACE ( 'NONE', ( #12193 ), #26819, .F. ) ;
#25525=VECTOR ( 'NONE', #4384, 39.37007874015748854 ) ;
#25527=CARTESIAN_POINT ( 'NONE',  ( 0.1574803149606299191, 0.9876813667277579700, 0.7893767492247204531 ) ) ;
#25556=ORIENTED_EDGE ( 'NONE', *, *, #8935, .F. ) ;
#25625=CARTESIAN_POINT ( 'NONE',  ( 0.1574803149606299191, 0.3740157480314960647, 0.9783464566929134243 ) ) ;
#25663=EDGE_LOOP ( 'NONE', ( #39370, #42027, #19371, #8418 ) ) ;
#25692=CARTESIAN_POINT ( 'NONE',  ( 0.000000000000000000, 0.000000000000000000, 0.000000000000000000 ) ) ;
#25706=CYLINDRICAL_SURFACE ( 'NONE', #30824, 0.3937007874015748254 ) ;
#25707=PLANE ( 'NONE',  #43322 ) ;
#25778=EDGE_CURVE ( 'NONE', #5864, #42441, #3980, .T. ) ;
#25797=CARTESIAN_POINT ( 'NONE',  ( 0.1126279540338993995, 0.3740157480314960647, 1.206847064312612128 ) ) ;
#25803=ORIENTED_EDGE ( 'NONE', *, *, #16570, .T. ) ;
#25818=CARTESIAN_POINT ( 'NONE',  ( 0.000000000000000000, 0.000000000000000000, 0.000000000000000000 ) ) ;
#25823=DIRECTION ( 'NONE',  ( 1.000000000000000000, 0.000000000000000000, -7.083454193571960199E-15 ) ) ;
#25824=AXIS2_PLACEMENT_3D ( 'NONE', #34975, #28745, #43309 ) ;
#25829=PLANE ( 'NONE',  #26757 ) ;
#25857=ORIENTED_EDGE ( 'NONE', *, *, #7616, .T. ) ;
#25877=DIRECTION ( 'NONE',  ( 1.000000000000000000, -5.472378587457090550E-15, 4.275490733183370330E-15 ) ) ;
#25888=DIRECTION ( 'NONE',  ( -1.000000000000000000, 0.000000000000000000, 7.047314121155780399E-15 ) ) ;
#25913=ORIENTED_EDGE ( 'NONE', *, *, #14079, .T. ) ;
#25952=DIRECTION ( 'NONE',  ( -5.159318851433039196E-16, -0.6156614753256609562, -0.7880107536067197938 ) ) ;
#25993=FACE_OUTER_BOUND ( 'NONE', #35522, .T. ) ;
#26002=LINE ( 'NONE', #29871, #39087 ) ;
#26021=ORIENTED_EDGE ( 'NONE', *, *, #22130, .F. ) ;
#26033=CARTESIAN_POINT ( 'NONE',  ( 0.000000000000000000, 0.4668427075568346574, -0.7022306805398661478 ) ) ;
#26057=DIRECTION ( 'NONE',  ( 7.083454193571959410E-15, 0.000000000000000000, 1.000000000000000000 ) ) ;
#26065=CARTESIAN_POINT ( 'NONE',  ( 0.000000000000000000, 0.6241017553149685870, 0.3240160679609074834 ) ) ;
#26151=ORIENTED_EDGE ( 'NONE', *, *, #14364, .F. ) ;
#26274=EDGE_CURVE ( 'NONE', #18566, #22479, #36361, .T. ) ;
#26292=AXIS2_PLACEMENT_3D ( 'NONE', #34593, #5584, #1743 ) ;
#26316=DIRECTION ( 'NONE',  ( -1.000000000000000000, 0.000000000000000000, 0.000000000000000000 ) ) ;
#26343=EDGE_LOOP ( 'NONE', ( #3173, #26367, #29498, #27969 ) ) ;
#26366=EDGE_CURVE ( 'NONE', #8447, #30077, #8703, .T. ) ;
#26367=ORIENTED_EDGE ( 'NONE', *, *, #29660, .F. ) ;
#26376=UNCERTAINTY_MEASURE_WITH_UNIT (LENGTH_MEASURE( 1.000000000000000082E-05 ), #21793, 'distance_accuracy_value', 'NONE') ;
#26395=DIRECTION ( 'NONE',  ( 0.000000000000000000, 0.000000000000000000, -1.000000000000000000 ) ) ;
#26546=DIRECTION ( 'NONE',  ( 0.000000000000000000, -0.6156614753256598460, -0.7880107536067206819 ) ) ;
#26614=ORIENTED_EDGE ( 'NONE', *, *, #16427, .F. ) ;
#26627=DIRECTION ( 'NONE',  ( -7.216634497304837451E-16, -0.6156614753256588468, -0.7880107536067216811 ) ) ;
#26685=CARTESIAN_POINT ( 'NONE',  ( 0.2362204724409449064, -0.5708661417322835607, 0.9783464566929134243 ) ) ;
#26691=ORIENTED_EDGE ( 'NONE', *, *, #47395, .T. ) ;
#26757=AXIS2_PLACEMENT_3D ( 'NONE', #40407, #160, #26546 ) ;
#26819=PLANE ( 'NONE',  #7223 ) ;
#26908=AXIS2_PLACEMENT_3D ( 'NONE', #27436, #41978, #46065 ) ;
#26921=AXIS2_PLACEMENT_3D ( 'NONE', #25818, #40397, #7583 ) ;
#26928=CARTESIAN_POINT ( 'NONE',  ( 0.2871444924769515628, 0.9382165298418956301, -1.070508272602716637 ) ) ;
#27025=( GEOMETRIC_REPRESENTATION_CONTEXT ( 3 ) GLOBAL_UNCERTAINTY_ASSIGNED_CONTEXT ( ( #2936 ) ) GLOBAL_UNIT_ASSIGNED_CONTEXT ( ( #19423, #19894, #30259 ) ) REPRESENTATION_CONTEXT ( 'NONE', 'WORKASPACE' ) ) ;
#27038=ORIENTED_EDGE ( 'NONE', *, *, #24684, .F. ) ;
#27041=ADVANCED_FACE ( 'NONE', ( #27320 ), #5708, .F. ) ;
#27109=EDGE_CURVE ( 'NONE', #43976, #32565, #30672, .T. ) ;
#27121=VERTEX_POINT ( 'NONE', #20324 ) ;
#27132=CARTESIAN_POINT ( 'NONE',  ( 0.000000000000000000, -0.5708661417322835607, 0.9783464566929134243 ) ) ;
#27191=VECTOR ( 'NONE', #24196, 39.37007874015748143 ) ;
#27211=VERTEX_POINT ( 'NONE', #24631 ) ;
#27231=CARTESIAN_POINT ( 'NONE',  ( 0.4736248074375818407, 1.488499961090669288, -0.3513258257898456138 ) ) ;
#27313=CARTESIAN_POINT ( 'NONE',  ( 0.1574803149606299191, 0.5288907983920094757, -0.7507079620615707549 ) ) ;
#27315=ADVANCED_FACE ( 'NONE', ( #17432 ), #32067, .F. ) ;
#27320=FACE_OUTER_BOUND ( 'NONE', #35216, .T. ) ;
#27361=AXIS2_PLACEMENT_3D ( 'NONE', #4273, #7418, #40229 ) ;
#27378=CARTESIAN_POINT ( 'NONE',  ( 0.2759478392031582961, -0.5708661417322835607, 1.214596435718460654 ) ) ;
#27428=EDGE_CURVE ( 'NONE', #183, #29781, #5979, .T. ) ;
#27436=CARTESIAN_POINT ( 'NONE',  ( 0.2871444924769515628, 0.9382165298418956301, -1.070508272602716637 ) ) ;
#27465=DIRECTION ( 'NONE',  ( -5.887603434621237738E-15, 0.7880107536067220142, -0.6156614753256581807 ) ) ;
#27480=ADVANCED_FACE ( 'NONE', ( #40401 ), #19071, .F. ) ;
#27516=CARTESIAN_POINT ( 'NONE',  ( 0.1574803149606299191, 0.1473293504822035527, -0.5595480905233944924 ) ) ;
#27536=CARTESIAN_POINT ( 'NONE',  ( 0.000000000000000000, 0.1473293504822035527, -0.9532488779249704836 ) ) ;
#27707=ORIENTED_EDGE ( 'NONE', *, *, #36274, .F. ) ;
#27723=EDGE_CURVE ( 'NONE', #21023, #24385, #45889, .T. ) ;
#27783=VECTOR ( 'NONE', #24180, 39.37007874015748854 ) ;
#27789=LINE ( 'NONE', #47314, #1780 ) ;
#27794=CARTESIAN_POINT ( 'NONE',  ( 0.04756641494945763188, 0.3740157480314960647, 1.120507485783946766 ) ) ;
#27889=AXIS2_PLACEMENT_3D ( 'NONE', #3803, #656, #39976 ) ;
#27905=ORIENTED_EDGE ( 'NONE', *, *, #23313, .T. ) ;
#27944=VECTOR ( 'NONE', #12565, 39.37007874015748143 ) ;
#27969=ORIENTED_EDGE ( 'NONE', *, *, #9854, .T. ) ;
#28018=LINE ( 'NONE', #42580, #22257 ) ;
#28046=DIRECTION ( 'NONE',  ( -1.000000000000000000, 0.000000000000000000, 0.000000000000000000 ) ) ;
#28093=DIRECTION ( 'NONE',  ( 0.000000000000000000, 1.000000000000000000, 0.000000000000000000 ) ) ;
#28097=ORIENTED_EDGE ( 'NONE', *, *, #8708, .F. ) ;
#28131=LINE ( 'NONE', #1997, #28280 ) ;
#28191=DIRECTION ( 'NONE',  ( -5.159318851433039196E-16, -0.6156614753256609562, -0.7880107536067197938 ) ) ;
#28280=VECTOR ( 'NONE', #42688, 39.37007874015748143 ) ;
#28362=FACE_OUTER_BOUND ( 'NONE', #24261, .T. ) ;
#28394=VECTOR ( 'NONE', #15707, 39.37007874015748854 ) ;
#28414=CIRCLE ( 'NONE', #31461, 0.02899999999999994596 ) ;
#28440=DIRECTION ( 'NONE',  ( 0.000000000000000000, 0.000000000000000000, -1.000000000000000000 ) ) ;
#28464=VECTOR ( 'NONE', #22624, 39.37007874015748854 ) ;
#28527=AXIS2_PLACEMENT_3D ( 'NONE', #36956, #37411, #25489 ) ;
#28572=CARTESIAN_POINT ( 'NONE',  ( 0.2759478392031617933, -0.5708661417322835607, 1.713085361781125915 ) ) ;
#28644=VERTEX_POINT ( 'NONE', #2918 ) ;
#28674=ADVANCED_FACE ( 'NONE', ( #28362 ), #13966, .T. ) ;
#28693=VERTEX_POINT ( 'NONE', #9675 ) ;
#28717=EDGE_CURVE ( 'NONE', #42931, #27211, #28131, .T. ) ;
#28723=DIRECTION ( 'NONE',  ( -0.000000000000000000, 0.6121968903568509868, 0.7907053606985360306 ) ) ;
#28733=DIRECTION ( 'NONE',  ( -1.000000000000000000, 0.000000000000000000, 0.000000000000000000 ) ) ;
#28741=AXIS2_PLACEMENT_3D ( 'NONE', #7673, #26627, #7915 ) ;
#28745=DIRECTION ( 'NONE',  ( 1.000000000000000000, 0.000000000000000000, 0.000000000000000000 ) ) ;
#28752=ORIENTED_EDGE ( 'NONE', *, *, #35518, .T. ) ;
#28771=ORIENTED_EDGE ( 'NONE', *, *, #9150, .F. ) ;
#28784=VERTEX_POINT ( 'NONE', #28853 ) ;
#28851=LINE ( 'NONE', #44069, #45169 ) ;
#28853=CARTESIAN_POINT ( 'NONE',  ( 0.1574803149606299191, 0.3740157480314960647, 0.9783464566929134243 ) ) ;
#28878=ORIENTED_EDGE ( 'NONE', *, *, #34470, .T. ) ;
#28886=ADVANCED_FACE ( 'NONE', ( #7249 ), #47263, .F. ) ;
#28896=VECTOR ( 'NONE', #44532, 39.37007874015748143 ) ;
#28978=DIRECTION ( 'NONE',  ( 0.000000000000000000, 0.000000000000000000, -1.000000000000000000 ) ) ;
#29044=DIRECTION ( 'NONE',  ( 7.047314121155781188E-15, 0.000000000000000000, 1.000000000000000000 ) ) ;
#29054=EDGE_CURVE ( 'NONE', #19538, #5864, #29088, .T. ) ;
#29088=CIRCLE ( 'NONE', #3797, 0.02900000000000052189 ) ;
#29140=AXIS2_PLACEMENT_3D ( 'NONE', #5964, #20583, #31404 ) ;
#29154=FACE_OUTER_BOUND ( 'NONE', #12407, .T. ) ;
#29172=PRODUCT ( 'Handle Arm Right', 'Handle Arm Right', '', ( #16382 ) ) ;
#29279=EDGE_LOOP ( 'NONE', ( #16199, #19620, #35786, #21248 ) ) ;
#29321=ORIENTED_EDGE ( 'NONE', *, *, #30826, .F. ) ;
#29458=DIRECTION ( 'NONE',  ( -2.943801717310650128E-16, 1.000000000000000000, 2.197428715927220134E-15 ) ) ;
#29474=DIRECTION ( 'NONE',  ( -1.000000000000000000, 0.000000000000000000, -6.938893903907220489E-15 ) ) ;
#29481=AXIS2_PLACEMENT_3D ( 'NONE', #34414, #842, #11903 ) ;
#29498=ORIENTED_EDGE ( 'NONE', *, *, #13085, .F. ) ;
#29518=PLANE ( 'NONE',  #1036 ) ;
#29549=ADVANCED_FACE ( 'NONE', ( #6949 ), #11046, .T. ) ;
#29569=DIRECTION ( 'NONE',  ( 7.083454193571959410E-15, 0.000000000000000000, 1.000000000000000000 ) ) ;
#29570=CIRCLE ( 'NONE', #11953, 0.1864803149606299448 ) ;
#29573=DIRECTION ( 'NONE',  ( -1.000000000000000000, 0.000000000000000000, 0.000000000000000000 ) ) ;
#29598=ADVANCED_FACE ( 'NONE', ( #11274 ), #7193, .T. ) ;
#29605=EDGE_LOOP ( 'NONE', ( #44369, #16597 ) ) ;
#29613=DIRECTION ( 'NONE',  ( 0.000000000000000000, 0.7907053606985359195, -0.6121968903568508757 ) ) ;
#29636=DIRECTION ( 'NONE',  ( -1.000000000000000000, 0.000000000000000000, 7.047314121155780399E-15 ) ) ;
#29640=CARTESIAN_POINT ( 'NONE',  ( 0.1574803149606299191, 0.000000000000000000, 0.2952755905511810774 ) ) ;
#29646=CARTESIAN_POINT ( 'NONE',  ( 0.1126279540338993995, 0.3740157480314960647, 1.206847064312612128 ) ) ;
#29659=ORIENTED_EDGE ( 'NONE', *, *, #8556, .T. ) ;
#29660=EDGE_CURVE ( 'NONE', #17962, #4180, #14156, .T. ) ;
#29681=DIRECTION ( 'NONE',  ( 7.703719777548939033E-31, -0.6156614753256599570, -0.7880107536067207930 ) ) ;
#29685=DIRECTION ( 'NONE',  ( 0.000000000000000000, -0.7880107536067206819, 0.6156614753256598460 ) ) ;
#29698=ORIENTED_EDGE ( 'NONE', *, *, #27109, .F. ) ;
#29722=CIRCLE ( 'NONE', #20501, 0.3912448816427545051 ) ;
#29781=VERTEX_POINT ( 'NONE', #457 ) ;
#29789=( LENGTH_UNIT ( ) NAMED_UNIT ( * ) SI_UNIT ( $, .METRE. ) ) ;
#29862=LINE ( 'NONE', #7522, #28464 ) ;
#29867=CARTESIAN_POINT ( 'NONE',  ( 0.1184675242425352465, -0.09842519685039370636, 2.185526306663015728 ) ) ;
#29871=CARTESIAN_POINT ( 'NONE',  ( 0.1184675242425285574, -0.5708661417322835607, 1.214596435718460654 ) ) ;
#29897=EDGE_LOOP ( 'NONE', ( #7976, #38835, #46253, #5247, #24887, #38946, #46840, #2085 ) ) ;
#29924=DIRECTION ( 'NONE',  ( 0.000000000000000000, 0.000000000000000000, -1.000000000000000000 ) ) ;
#29932=DIRECTION ( 'NONE',  ( -6.938893903907234689E-15, 0.000000000000000000, 1.000000000000000000 ) ) ;
#29981=ORIENTED_EDGE ( 'NONE', *, *, #5862, .T. ) ;
#30019=VECTOR ( 'NONE', #154, 39.37007874015748143 ) ;
#30077=VERTEX_POINT ( 'NONE', #3551 ) ;
#30129=ORIENTED_EDGE ( 'NONE', *, *, #20826, .F. ) ;
#30132=LINE ( 'NONE', #8508, #33601 ) ;
#30139=DIRECTION ( 'NONE',  ( 0.000000000000000000, 1.000000000000000000, 0.000000000000000000 ) ) ;
#30227=EDGE_LOOP ( 'NONE', ( #39381, #11630, #8806, #10834 ) ) ;
#30259=( NAMED_UNIT ( * ) SI_UNIT ( $, .STERADIAN. ) SOLID_ANGLE_UNIT ( ) ) ;
#30313=AXIS2_PLACEMENT_3D ( 'NONE', #27536, #42087, #12669 ) ;
#30350=AXIS2_PLACEMENT_3D ( 'NONE', #4223, #19574, #22693 ) ;
#30357=ADVANCED_FACE ( 'NONE', ( #19086 ), #622, .F. ) ;
#30362=ORIENTED_EDGE ( 'NONE', *, *, #19032, .T. ) ;
#30501=VERTEX_POINT ( 'NONE', #9268 ) ;
#30520=ORIENTED_EDGE ( 'NONE', *, *, #28717, .T. ) ;
#30532=LINE ( 'NONE', #1016, #24640 ) ;
#30585=DIRECTION ( 'NONE',  ( -1.000000000000000000, 0.000000000000000000, -7.047314121155770932E-15 ) ) ;
#30624=LINE ( 'NONE', #22211, #15791 ) ;
#30672=LINE ( 'NONE', #19853, #12892 ) ;
#30694=DIRECTION ( 'NONE',  ( 0.000000000000000000, 0.2432573283306889156, -0.9699617890481125881 ) ) ;
#30709=ORIENTED_EDGE ( 'NONE', *, *, #23549, .F. ) ;
#30746=ORIENTED_EDGE ( 'NONE', *, *, #20407, .T. ) ;
#30757=VECTOR ( 'NONE', #38263, 39.37007874015748854 ) ;
#30758=EDGE_CURVE ( 'NONE', #43422, #183, #18107, .T. ) ;
#30760=CIRCLE ( 'NONE', #26921, 0.2952755905511810774 ) ;
#30780=AXIS2_PLACEMENT_3D ( 'NONE', #3463, #18317, #9781 ) ;
#30795=CARTESIAN_POINT ( 'NONE',  ( 0.1574803149606299191, 0.1473293504822035527, -0.5595480905233944924 ) ) ;
#30811=DIRECTION ( 'NONE',  ( 0.000000000000000000, 0.6156614753256598460, 0.7880107536067206819 ) ) ;
#30824=AXIS2_PLACEMENT_3D ( 'NONE', #44342, #29573, #15386 ) ;
#30826=EDGE_CURVE ( 'NONE', #4180, #31929, #7080, .T. ) ;
#30873=AXIS2_PLACEMENT_3D ( 'NONE', #10260, #6404, #21016 ) ;
#30905=ORIENTED_EDGE ( 'NONE', *, *, #4470, .F. ) ;
#30930=DIRECTION ( 'NONE',  ( -1.000000000000000000, -5.411399086424350389E-15, 4.197754538034584604E-15 ) ) ;
#30958=( GEOMETRIC_REPRESENTATION_CONTEXT ( 3 ) GLOBAL_UNCERTAINTY_ASSIGNED_CONTEXT ( ( #26376 ) ) GLOBAL_UNIT_ASSIGNED_CONTEXT ( ( #21793, #37100, #44510 ) ) REPRESENTATION_CONTEXT ( 'NONE', 'WORKASPACE' ) ) ;
#30969=PLANE ( 'NONE',  #46754 ) ;
#30970=ADVANCED_FACE ( 'NONE', ( #8186 ), #45068, .T. ) ;
#30994=DIRECTION ( 'NONE',  ( 0.000000000000000000, -0.7880107536067211260, 0.6156614753256591799 ) ) ;
#30997=ORIENTED_EDGE ( 'NONE', *, *, #20407, .F. ) ;
#31000=DIRECTION ( 'NONE',  ( -0.6018150231520440485, 0.000000000000000000, -0.7986355100472960489 ) ) ;
#31019=AXIS2_PLACEMENT_3D ( 'NONE', #9634, #46503, #28093 ) ;
#31058=AXIS2_PLACEMENT_3D ( 'NONE', #46873, #20991, #35640 ) ;
#31065=ORIENTED_EDGE ( 'NONE', *, *, #35715, .T. ) ;
#31090=DIRECTION ( 'NONE',  ( 0.000000000000000000, 0.7880107536067213481, -0.6156614753256589578 ) ) ;
#31132=DIRECTION ( 'NONE',  ( 1.000000000000000000, 0.000000000000000000, 0.000000000000000000 ) ) ;
#31147=EDGE_CURVE ( 'NONE', #35620, #27211, #13066, .T. ) ;
#31162=DIRECTION ( 'NONE',  ( 5.411399086424348811E-15, -1.000000000000000000, 0.000000000000000000 ) ) ;
#31214=ORIENTED_EDGE ( 'NONE', *, *, #14520, .T. ) ;
#31221=AXIS2_PLACEMENT_3D ( 'NONE', #4625, #7525, #18784 ) ;
#31238=CARTESIAN_POINT ( 'NONE',  ( -0.4955489724641236604, 0.000000000000000000, 0.3997690233743834698 ) ) ;
#31250=ORIENTED_EDGE ( 'NONE', *, *, #40796, .F. ) ;
#31284=CARTESIAN_POINT ( 'NONE',  ( 0.3161444924769420961, -1.730062351173306868E-15, 1.351672847932125986E-15 ) ) ;
#31315=DIRECTION ( 'NONE',  ( 1.000000000000000000, 0.000000000000000000, 2.048823632034775047E-14 ) ) ;
#31384=AXIS2_PLACEMENT_3D ( 'NONE', #22405, #15478, #32990 ) ;
#31404=DIRECTION ( 'NONE',  ( -0.7986355100472968260, 0.000000000000000000, 0.6018150231520429383 ) ) ;
#31460=DIRECTION ( 'NONE',  ( 0.8191520442889949072, -0.4519843998600416302, 0.3531289150159167556 ) ) ;
#31461=AXIS2_PLACEMENT_3D ( 'NONE', #20032, #1820, #31090 ) ;
#31487=DIRECTION ( 'NONE',  ( -3.662381193211854913E-16, 1.000000000000000000, 2.355041373848520102E-15 ) ) ;
#31489=LINE ( 'NONE', #23107, #188 ) ;
#31552=FACE_OUTER_BOUND ( 'NONE', #4454, .T. ) ;
#31556=ORIENTED_EDGE ( 'NONE', *, *, #24615, .T. ) ;
#31603=ORIENTED_EDGE ( 'NONE', *, *, #9816, .T. ) ;
#31607=CYLINDRICAL_SURFACE ( 'NONE', #30873, 0.5708661417322835607 ) ;
#31611=LINE ( 'NONE', #16973, #24579 ) ;
#31656=LINE ( 'NONE', #10306, #38567 ) ;
#31671=EDGE_CURVE ( 'NONE', #32150, #712, #19616, .T. ) ;
#31704=CARTESIAN_POINT ( 'NONE',  ( 0.3161444924769515885, 0.4457451269443646336, -1.671447902550338815 ) ) ;
#31728=DIRECTION ( 'NONE',  ( -6.944548107256197364E-15, -0.7880107536067206819, 0.6156614753256598460 ) ) ;
#31733=ORIENTED_EDGE ( 'NONE', *, *, #32553, .T. ) ;
#31751=CLOSED_SHELL ( 'NONE', ( #47293, #4972, #18448, #29549, #1903, #16780, #28674, #6920, #17527, #15873, #30970, #19195, #36087, #14533, #9916, #32141, #8016, #6326, #27315, #5748, #33139, #41636, #3575, #15636, #39601, #14254, #39921, #9485, #27480, #44828, #28886, #7321, #36532, #3919, #37331, #25520, #5570, #32601, #33189, #730, #38632, #23444, #16646, #24617, #45380, #41241, #43922, #21719, #27041, #9864, #8039, #29598, #9323, #38538, #30357 ) ) ;
#31815=ORIENTED_EDGE ( 'NONE', *, *, #47080, .T. ) ;
#31827=EDGE_CURVE ( 'NONE', #18734, #28693, #28018, .T. ) ;
#31832=VECTOR ( 'NONE', #45151, 39.37007874015748143 ) ;
#31845=DIRECTION ( 'NONE',  ( 7.542275982507857147E-17, -0.6156614753256598460, -0.7880107536067206819 ) ) ;
#31870=CARTESIAN_POINT ( 'NONE',  ( 0.4736248074375574713, 1.975221432870720495, -0.9622519263226653186 ) ) ;
#31877=VECTOR ( 'NONE', #4469, 39.37007874015748143 ) ;
#31929=VERTEX_POINT ( 'NONE', #14614 ) ;
#31963=CYLINDRICAL_SURFACE ( 'NONE', #19677, 0.4724409448818896462 ) ;
#31982=DIRECTION ( 'NONE',  ( 1.000000000000000000, 0.000000000000000000, -4.710082747697005495E-15 ) ) ;
#31990=DIRECTION ( 'NONE',  ( 0.000000000000000000, 0.000000000000000000, 1.000000000000000000 ) ) ;
#32026=CARTESIAN_POINT ( 'NONE',  ( 0.000000000000000000, 0.3740157480314960647, 0.9783464566929134243 ) ) ;
#32067=CYLINDRICAL_SURFACE ( 'NONE', #7515, 0.02900000000000001882 ) ;
#32141=ADVANCED_FACE ( 'NONE', ( #31552 ), #24345, .T. ) ;
#32150=VERTEX_POINT ( 'NONE', #2515 ) ;
#32158=EDGE_LOOP ( 'NONE', ( #21728, #6704, #10097, #3369 ) ) ;
#32159=CARTESIAN_POINT ( 'NONE',  ( -0.3115983495410063475, 0.1719309546946380107, -0.1343271836544986386 ) ) ;
#32225=CIRCLE ( 'NONE', #3866, 0.1864803149606298061 ) ;
#32248=VECTOR ( 'NONE', #44413, 39.37007874015748143 ) ;
#32266=VERTEX_POINT ( 'NONE', #2053 ) ;
#32294=ORIENTED_EDGE ( 'NONE', *, *, #44681, .T. ) ;
#32528=EDGE_LOOP ( 'NONE', ( #5117, #32861, #4197, #17118 ) ) ;
#32553=EDGE_CURVE ( 'NONE', #18566, #6306, #12918, .T. ) ;
#32561=CARTESIAN_POINT ( 'NONE',  ( 0.02847999302535491814, 0.6072747502901004735, -0.8119482170283445210 ) ) ;
#32565=VERTEX_POINT ( 'NONE', #9548 ) ;
#32601=ADVANCED_FACE ( 'NONE', ( #9782, #24171 ), #20549, .T. ) ;
#32618=ORIENTED_EDGE ( 'NONE', *, *, #31827, .T. ) ;
#32652=DIRECTION ( 'NONE',  ( 0.000000000000000000, 0.000000000000000000, 1.000000000000000000 ) ) ;
#32710=CARTESIAN_POINT ( 'NONE',  ( -0.4955489724641236604, -0.5708661417322835607, 0.3997690233743834698 ) ) ;
#32818=DIRECTION ( 'NONE',  ( -1.000000000000000000, 0.000000000000000000, 0.000000000000000000 ) ) ;
#32843=ORIENTED_EDGE ( 'NONE', *, *, #38703, .T. ) ;
#32861=ORIENTED_EDGE ( 'NONE', *, *, #36274, .T. ) ;
#32862=ORIENTED_EDGE ( 'NONE', *, *, #42616, .F. ) ;
#32881=CARTESIAN_POINT ( 'NONE',  ( 0.1184675242425285574, -0.5708661417322835607, 1.224299699984019663 ) ) ;
#32950=CIRCLE ( 'NONE', #33714, 0.5905511811023621549 ) ;
#32971=DIRECTION ( 'NONE',  ( -2.038787975192215258E-30, -1.000000000000000000, -2.891205793294680298E-16 ) ) ;
#32974=ORIENTED_EDGE ( 'NONE', *, *, #26366, .F. ) ;
#32990=DIRECTION ( 'NONE',  ( 0.000000000000000000, -1.406820448837680035E-16, -1.000000000000000000 ) ) ;
#32996=LINE ( 'NONE', #25797, #34843 ) ;
#33009=DIRECTION ( 'NONE',  ( 0.000000000000000000, -0.7880107536067206819, 0.6156614753256598460 ) ) ;
#33030=LINE ( 'NONE', #42808, #17754 ) ;
#33139=ADVANCED_FACE ( 'NONE', ( #17547 ), #12802, .F. ) ;
#33186=LINE ( 'NONE', #32710, #20830 ) ;
#33189=ADVANCED_FACE ( 'NONE', ( #24721 ), #39321, .T. ) ;
#33199=EDGE_CURVE ( 'NONE', #34892, #22479, #18721, .T. ) ;
#33210=CARTESIAN_POINT ( 'NONE',  ( 0.1574803149606299191, -0.5708661417322835607, 0.9783464566929134243 ) ) ;
#33382=AXIS2_PLACEMENT_3D ( 'NONE', #31238, #38871, #6035 ) ;
#33393=ORIENTED_EDGE ( 'NONE', *, *, #45212, .F. ) ;
#33407=EDGE_LOOP ( 'NONE', ( #26021, #40364, #19747, #23770 ) ) ;
#33437=DIRECTION ( 'NONE',  ( -2.114720919224289611E-16, 1.000000000000000000, 0.000000000000000000 ) ) ;
#33555=VERTEX_POINT ( 'NONE', #1213 ) ;
#33562=CARTESIAN_POINT ( 'NONE',  ( 0.3161444924769511999, 0.9382165298418956301, -1.070508272602716637 ) ) ;
#33601=VECTOR ( 'NONE', #23608, 39.37007874015748143 ) ;
#33643=VECTOR ( 'NONE', #18097, 39.37007874015748854 ) ;
#33648=CARTESIAN_POINT ( 'NONE',  ( 0.2362204724409449064, -0.5708661417322835607, 0.9783464566929134243 ) ) ;
#33699=EDGE_CURVE ( 'NONE', #43030, #38536, #33030, .T. ) ;
#33714=AXIS2_PLACEMENT_3D ( 'NONE', #22765, #28046, #16998 ) ;
#33743=DIRECTION ( 'NONE',  ( 0.000000000000000000, 0.000000000000000000, 1.000000000000000000 ) ) ;
#33759=ORIENTED_EDGE ( 'NONE', *, *, #18368, .T. ) ;
#33791=CARTESIAN_POINT ( 'NONE',  ( 0.3108999017613323090, 0.9251089822459547252, -1.060267534067256046 ) ) ;
#33823=CYLINDRICAL_SURFACE ( 'NONE', #43614, 0.1864803149606299171 ) ;
#33833=DIMENSIONAL_EXPONENTS ( 1.000000000000000000, 0.000000000000000000, 0.000000000000000000, 0.000000000000000000, 0.000000000000000000, 0.000000000000000000, 0.000000000000000000 ) ;
#33891=FACE_OUTER_BOUND ( 'NONE', #12451, .T. ) ;
#33901=VECTOR ( 'NONE', #44882, 39.37007874015748143 ) ;
#33908=CARTESIAN_POINT ( 'NONE',  ( 0.1733357866104492107, -0.5708661417322835607, 1.025733466389925352 ) ) ;
#33916=CARTESIAN_POINT ( 'NONE',  ( 0.4736248074375716821, -2.599213366583078641E-15, 2.030728043535499967E-15 ) ) ;
#33925=DIRECTION ( 'NONE',  ( 0.7986355100472766200, 1.652401737524974224E-15, -0.6018150231520698057 ) ) ;
#33949=CARTESIAN_POINT ( 'NONE',  ( 0.000000000000000000, 0.5288907983920094757, -0.7507079620615707549 ) ) ;
#33982=DIRECTION ( 'NONE',  ( 0.000000000000000000, -0.7880107536067199048, 0.6156614753256609562 ) ) ;
#34033=ORIENTED_EDGE ( 'NONE', *, *, #4470, .T. ) ;
#34135=FACE_OUTER_BOUND ( 'NONE', #18937, .T. ) ;
#34142=CARTESIAN_POINT ( 'NONE',  ( 0.1627249056762490320, 1.099487083487566963, -0.04739565599252346800 ) ) ;
#34163=AXIS2_PLACEMENT_3D ( 'NONE', #41525, #23829, #16863 ) ;
#34207=PLANE ( 'NONE',  #21551 ) ;
#34212=CARTESIAN_POINT ( 'NONE',  ( 0.1574803149606299191, 0.3740157480314960647, 0.9783464566929134243 ) ) ;
#34265=CARTESIAN_POINT ( 'NONE',  ( 0.3161444924769535869, 1.205832402325950792, -1.129708666049259902 ) ) ;
#34327=DIRECTION ( 'NONE',  ( 3.074932031758790220E-16, -1.000000000000000000, -7.235709728040729085E-17 ) ) ;
#34372=EDGE_CURVE ( 'NONE', #18734, #9939, #37591, .T. ) ;
#34414=CARTESIAN_POINT ( 'NONE',  ( -0.3697796008031323245, 0.000000000000000000, 0.3049950039803606128 ) ) ;
#34470=EDGE_CURVE ( 'NONE', #36104, #40667, #39003, .T. ) ;
#34574=DIRECTION ( 'NONE',  ( -6.938893903907234689E-15, 0.000000000000000000, 1.000000000000000000 ) ) ;
#34593=CARTESIAN_POINT ( 'NONE',  ( 0.2759478392031617933, -0.09842519685039370636, 1.713085361781127913 ) ) ;
#34638=CIRCLE ( 'NONE', #38453, 0.3937007874015747699 ) ;
#34652=EDGE_CURVE ( 'NONE', #32565, #7704, #34638, .T. ) ;
#34661=LINE ( 'NONE', #24111, #3930 ) ;
#34674=LINE ( 'NONE', #34212, #33643 ) ;
#34789=ORIENTED_EDGE ( 'NONE', *, *, #11426, .F. ) ;
#34818=AXIS2_PLACEMENT_3D ( 'NONE', #6019, #2426, #34821 ) ;
#34821=DIRECTION ( 'NONE',  ( 1.000000000000000000, -9.297927578135879519E-16, 0.000000000000000000 ) ) ;
#34831=LINE ( 'NONE', #20652, #11136 ) ;
#34843=VECTOR ( 'NONE', #40602, 39.37007874015748143 ) ;
#34852=DIRECTION ( 'NONE',  ( 1.000000000000000000, 3.662381193212024518E-16, -7.324762386424049233E-15 ) ) ;
#34892=VERTEX_POINT ( 'NONE', #15717 ) ;
#34914=VERTEX_POINT ( 'NONE', #41771 ) ;
#34933=ORIENTED_EDGE ( 'NONE', *, *, #45147, .F. ) ;
#34943=VERTEX_POINT ( 'NONE', #5367 ) ;
#34958=DIRECTION ( 'NONE',  ( -1.000000000000000000, 0.000000000000000000, 7.051687499798870116E-15 ) ) ;
#34962=FACE_OUTER_BOUND ( 'NONE', #25249, .T. ) ;
#34975=CARTESIAN_POINT ( 'NONE',  ( 0.000000000000000000, 0.000000000000000000, 0.000000000000000000 ) ) ;
#35032=DIRECTION ( 'NONE',  ( -1.000000000000000000, 0.000000000000000000, -7.051687499798870116E-15 ) ) ;
#35049=CARTESIAN_POINT ( 'NONE',  ( 0.4736248074375850603, 1.357244529069700612, -1.397888825503269761 ) ) ;
#35051=DIRECTION ( 'NONE',  ( 0.000000000000000000, -0.6156614753256598460, -0.7880107536067206819 ) ) ;
#35106=ORIENTED_EDGE ( 'NONE', *, *, #9368, .T. ) ;
#35163=AXIS2_PLACEMENT_3D ( 'NONE', #8442, #11588, #19704 ) ;
#35167=ORIENTED_EDGE ( 'NONE', *, *, #9368, .F. ) ;
#35204=ORIENTED_EDGE ( 'NONE', *, *, #46184, .F. ) ;
#35216=EDGE_LOOP ( 'NONE', ( #38965, #8431, #21661, #39189 ) ) ;
#35237=CARTESIAN_POINT ( 'NONE',  ( 0.4451448144122268080, 1.417321315443419438, -0.2957149730314338476 ) ) ;
#35279=VERTEX_POINT ( 'NONE', #22580 ) ;
#35299=DIRECTION ( 'NONE',  ( 1.000000000000000000, -5.464378949326940770E-15, 4.275490733183370330E-15 ) ) ;
#35415=VECTOR ( 'NONE', #35032, 39.37007874015748143 ) ;
#35477=DIRECTION ( 'NONE',  ( 0.000000000000000000, 6.980778575359379259E-17, -1.000000000000000000 ) ) ;
#35518=EDGE_CURVE ( 'NONE', #10419, #21057, #16582, .T. ) ;
#35522=EDGE_LOOP ( 'NONE', ( #2761, #3572, #7656, #7221, #7672, #36813, #35167, #11660 ) ) ;
#35620=VERTEX_POINT ( 'NONE', #11971 ) ;
#35640=DIRECTION ( 'NONE',  ( 0.000000000000000000, 6.980778575359379259E-17, -1.000000000000000000 ) ) ;
#35700=ORIENTED_EDGE ( 'NONE', *, *, #44681, .F. ) ;
#35715=EDGE_CURVE ( 'NONE', #36104, #34892, #4741, .T. ) ;
#35777=CARTESIAN_POINT ( 'NONE',  ( 0.08946752424252854552, 0.3740157480314960647, 1.224299699984021661 ) ) ;
#35786=ORIENTED_EDGE ( 'NONE', *, *, #38043, .T. ) ;
#35849=EDGE_LOOP ( 'NONE', ( #23266, #22987 ) ) ;
#35855=EDGE_CURVE ( 'NONE', #10419, #12883, #7896, .T. ) ;
#35866=VECTOR ( 'NONE', #12175, 39.37007874015748143 ) ;
#35921=EDGE_CURVE ( 'NONE', #27211, #712, #27789, .T. ) ;
#35986=AXIS2_PLACEMENT_3D ( 'NONE', #22732, #2675, #18891 ) ;
#36030=AXIS2_PLACEMENT_3D ( 'NONE', #9252, #39172, #31315 ) ;
#36035=VECTOR ( 'NONE', #28191, 39.37007874015748143 ) ;
#36039=CYLINDRICAL_SURFACE ( 'NONE', #16876, 0.02900000000000000147 ) ;
#36046=ORIENTED_EDGE ( 'NONE', *, *, #23757, .F. ) ;
#36047=EDGE_CURVE ( 'NONE', #34943, #34914, #36764, .T. ) ;
#36060=VECTOR ( 'NONE', #14145, 39.37007874015748143 ) ;
#36087=ADVANCED_FACE ( 'NONE', ( #34135 ), #1265, .T. ) ;
#36104=VERTEX_POINT ( 'NONE', #42227 ) ;
#36109=CIRCLE ( 'NONE', #21556, 0.1864803149606298061 ) ;
#36117=ORIENTED_EDGE ( 'NONE', *, *, #6428, .F. ) ;
#36130=DIRECTION ( 'NONE',  ( 8.117793622096712470E-16, -0.6156614753256580697, -0.7880107536067222362 ) ) ;
#36237=ORIENTED_EDGE ( 'NONE', *, *, #7036, .F. ) ;
#36258=DIRECTION ( 'NONE',  ( 0.7986355100472770641, 0.000000000000000000, -0.6018150231520690285 ) ) ;
#36269=EDGE_CURVE ( 'NONE', #12883, #10419, #14787, .T. ) ;
#36274=EDGE_CURVE ( 'NONE', #44909, #6306, #17073, .T. ) ;
#36327=ORIENTED_EDGE ( 'NONE', *, *, #23644, .T. ) ;
#36341=PLANE ( 'NONE',  #31384 ) ;
#36361=CIRCLE ( 'NONE', #1118, 0.02900000000000052189 ) ;
#36375=ORIENTED_EDGE ( 'NONE', *, *, #20826, .T. ) ;
#36385=CIRCLE ( 'NONE', #37147, 0.2952755905511810774 ) ;
#36409=LINE ( 'NONE', #3566, #44011 ) ;
#36410=CARTESIAN_POINT ( 'NONE',  ( 0.4736248074375795647, 1.690605217543005745, -0.5092277576975118292 ) ) ;
#36532=ADVANCED_FACE ( 'NONE', ( #14671 ), #25706, .F. ) ;
#36544=DIRECTION ( 'NONE',  ( -4.275490733183370330E-15, 0.000000000000000000, 1.000000000000000000 ) ) ;
#36636=EDGE_CURVE ( 'NONE', #30501, #5626, #11086, .T. ) ;
#36709=DIRECTION ( 'NONE',  ( 0.000000000000000000, -0.7880107536067197938, 0.6156614753256609562 ) ) ;
#36710=DIRECTION ( 'NONE',  ( -0.5735764363510409414, -0.6455006197386570221, 0.5043203561029929727 ) ) ;
#36739=ORIENTED_EDGE ( 'NONE', *, *, #18830, .T. ) ;
#36750=ORIENTED_EDGE ( 'NONE', *, *, #15768, .F. ) ;
#36764=LINE ( 'NONE', #33908, #38519 ) ;
#36781=LINE ( 'NONE', #96, #2368 ) ;
#36784=ORIENTED_EDGE ( 'NONE', *, *, #36269, .T. ) ;
#36796=CIRCLE ( 'NONE', #5401, 0.5708661417322835607 ) ;
#36813=ORIENTED_EDGE ( 'NONE', *, *, #38043, .F. ) ;
#36819=CARTESIAN_POINT ( 'NONE',  ( 0.4736248074375850603, 1.357244529069700612, -1.397888825503269761 ) ) ;
#36844=VERTEX_POINT ( 'NONE', #42632 ) ;
#36847=ORIENTED_EDGE ( 'NONE', *, *, #20684, .F. ) ;
#36864=LINE ( 'NONE', #25625, #31877 ) ;
#36875=FACE_BOUND ( 'NONE', #29605, .T. ) ;
#36896=VERTEX_POINT ( 'NONE', #6751 ) ;
#36924=VERTEX_POINT ( 'NONE', #6993 ) ;
#36956=CARTESIAN_POINT ( 'NONE',  ( 0.1574803149606299191, 0.1473293504822035527, -0.9532488779249704836 ) ) ;
#36978=PLANE ( 'NONE',  #8352 ) ;
#37011=DIRECTION ( 'NONE',  ( -1.000000000000000000, 0.000000000000000000, 0.000000000000000000 ) ) ;
#37037=ORIENTED_EDGE ( 'NONE', *, *, #21530, .F. ) ;
#37100=( NAMED_UNIT ( * ) PLANE_ANGLE_UNIT ( ) SI_UNIT ( $, .RADIAN. ) ) ;
#37147=AXIS2_PLACEMENT_3D ( 'NONE', #44327, #19173, #26395 ) ;
#37331=ADVANCED_FACE ( 'NONE', ( #21559 ), #29518, .F. ) ;
#37351=ORIENTED_EDGE ( 'NONE', *, *, #2146, .T. ) ;
#37357=CIRCLE ( 'NONE', #3706, 0.2952755905511810774 ) ;
#37375=CYLINDRICAL_SURFACE ( 'NONE', #28741, 0.1864803149606298893 ) ;
#37411=DIRECTION ( 'NONE',  ( -1.000000000000000000, 0.000000000000000000, 0.000000000000000000 ) ) ;
#37478=DIRECTION ( 'NONE',  ( 7.047314121155781188E-15, 0.000000000000000000, 1.000000000000000000 ) ) ;
#37545=EDGE_CURVE ( 'NONE', #22479, #40667, #13047, .T. ) ;
#37581=ORIENTED_EDGE ( 'NONE', *, *, #21530, .T. ) ;
#37591=LINE ( 'NONE', #19379, #17010 ) ;
#37631=ORIENTED_EDGE ( 'NONE', *, *, #24906, .F. ) ;
#37650=DIRECTION ( 'NONE',  ( -1.000000000000000000, 0.000000000000000000, 6.123233995736769734E-17 ) ) ;
#37654=ORIENTED_EDGE ( 'NONE', *, *, #18826, .F. ) ;
#37657=CARTESIAN_POINT ( 'NONE',  ( 0.1864803149606299171, 1.086379535891623949, -0.03715491745706173132 ) ) ;
#37711=CIRCLE ( 'NONE', #21710, 0.7874015748031496509 ) ;
#37729=ORIENTED_EDGE ( 'NONE', *, *, #14079, .F. ) ;
#37756=ORIENTED_EDGE ( 'NONE', *, *, #27723, .F. ) ;
#37758=ORIENTED_EDGE ( 'NONE', *, *, #16832, .T. ) ;
#37794=CARTESIAN_POINT ( 'NONE',  ( 0.1574803149606299191, 0.000000000000000000, 0.000000000000000000 ) ) ;
#37906=VECTOR ( 'NONE', #17239, 39.37007874015748143 ) ;
#37989=EDGE_LOOP ( 'NONE', ( #37756, #34933, #30905, #44553 ) ) ;
#38029=DIRECTION ( 'NONE',  ( -1.000000000000000000, 0.000000000000000000, 0.000000000000000000 ) ) ;
#38033=EDGE_CURVE ( 'NONE', #28644, #18361, #41689, .T. ) ;
#38043=EDGE_CURVE ( 'NONE', #42894, #28693, #41158, .T. ) ;
#38150=ORIENTED_EDGE ( 'NONE', *, *, #3053, .T. ) ;
#38197=ORIENTED_EDGE ( 'NONE', *, *, #30826, .T. ) ;
#38211=DIRECTION ( 'NONE',  ( 5.724375810226159034E-16, 0.6156614753256599570, 0.7880107536067207930 ) ) ;
#38263=DIRECTION ( 'NONE',  ( -0.6018150231520440485, 0.000000000000000000, -0.7986355100472960489 ) ) ;
#38373=CARTESIAN_POINT ( 'NONE',  ( 0.4736248074375858375, -0.09842519685039370636, 1.870565676741759775 ) ) ;
#38386=AXIS2_PLACEMENT_3D ( 'NONE', #18153, #28733, #28978 ) ;
#38393=DIRECTION ( 'NONE',  ( -4.825174235490821143E-17, -0.6156614753256592909, -0.7880107536067212370 ) ) ;
#38453=AXIS2_PLACEMENT_3D ( 'NONE', #13793, #13342, #28440 ) ;
#38456=DIRECTION ( 'NONE',  ( -1.739631066775710943E-15, -2.197428715927213823E-15, 1.000000000000000000 ) ) ;
#38462=VECTOR ( 'NONE', #6771, 39.37007874015748854 ) ;
#38501=EDGE_LOOP ( 'NONE', ( #26614, #6254, #21175, #39730, #22481 ) ) ;
#38519=VECTOR ( 'NONE', #8460, 39.37007874015748854 ) ;
#38536=VERTEX_POINT ( 'NONE', #26065 ) ;
#38538=ADVANCED_FACE ( 'NONE', ( #40872 ), #18618, .F. ) ;
#38567=VECTOR ( 'NONE', #35477, 39.37007874015748143 ) ;
#38568=LINE ( 'NONE', #12479, #27191 ) ;
#38622=AXIS2_PLACEMENT_3D ( 'NONE', #39079, #10107, #20876 ) ;
#38625=EDGE_CURVE ( 'NONE', #45189, #43030, #29570, .T. ) ;
#38630=LINE ( 'NONE', #35049, #18020 ) ;
#38632=ADVANCED_FACE ( 'NONE', ( #15053 ), #4448, .F. ) ;
#38666=DIRECTION ( 'NONE',  ( -1.000000000000000000, 0.000000000000000000, 0.000000000000000000 ) ) ;
#38691=ORIENTED_EDGE ( 'NONE', *, *, #16832, .F. ) ;
#38703=EDGE_CURVE ( 'NONE', #24486, #36924, #30624, .T. ) ;
#38740=LINE ( 'NONE', #1831, #30757 ) ;
#38777=DIRECTION ( 'NONE',  ( -1.000000000000000000, 0.000000000000000000, 0.000000000000000000 ) ) ;
#38805=FACE_OUTER_BOUND ( 'NONE', #24941, .T. ) ;
#38807=DIRECTION ( 'NONE',  ( 1.000000000000000000, 5.372880794957870593E-15, -4.197754538034579871E-15 ) ) ;
#38835=ORIENTED_EDGE ( 'NONE', *, *, #11792, .T. ) ;
#38871=DIRECTION ( 'NONE',  ( 0.7986355100472960489, 0.000000000000000000, -0.6018150231520441595 ) ) ;
#38939=FACE_OUTER_BOUND ( 'NONE', #32158, .T. ) ;
#38946=ORIENTED_EDGE ( 'NONE', *, *, #34372, .F. ) ;
#38965=ORIENTED_EDGE ( 'NONE', *, *, #23313, .F. ) ;
#38987=CARTESIAN_POINT ( 'NONE',  ( 0.1574803149606299191, 0.5360961046428496246, -0.7563373642699310340 ) ) ;
#39003=LINE ( 'NONE', #32561, #27783 ) ;
#39004=DIRECTION ( 'NONE',  ( 2.943801717310650128E-16, -1.000000000000000000, -2.355041373848520102E-15 ) ) ;
#39059=VECTOR ( 'NONE', #23842, 39.37007874015748854 ) ;
#39074=PLANE ( 'NONE',  #31019 ) ;
#39079=CARTESIAN_POINT ( 'NONE',  ( 0.08946752424252854552, 0.3740157480314960647, 1.224299699984021661 ) ) ;
#39087=VECTOR ( 'NONE', #11160, 39.37007874015748143 ) ;
#39127=AXIS2_PLACEMENT_3D ( 'NONE', #9769, #46639, #24156 ) ;
#39135=VECTOR ( 'NONE', #20020, 39.37007874015748143 ) ;
#39153=FACE_OUTER_BOUND ( 'NONE', #26343, .T. ) ;
#39172=DIRECTION ( 'NONE',  ( -4.357234436330879339E-15, 0.9771240687918565371, 0.2126700594527759225 ) ) ;
#39189=ORIENTED_EDGE ( 'NONE', *, *, #9150, .T. ) ;
#39267=EDGE_CURVE ( 'NONE', #8850, #580, #15032, .T. ) ;
#39276=DIRECTION ( 'NONE',  ( -7.051687499798870116E-15, -1.406820448837680035E-16, -1.000000000000000000 ) ) ;
#39321=PLANE ( 'NONE',  #40746 ) ;
#39352=LINE ( 'NONE', #21388, #17792 ) ;
#39370=ORIENTED_EDGE ( 'NONE', *, *, #21541, .T. ) ;
#39376=CARTESIAN_POINT ( 'NONE',  ( 0.08946752424252854552, 0.3740157480314960647, 1.224299699984021661 ) ) ;
#39381=ORIENTED_EDGE ( 'NONE', *, *, #12899, .T. ) ;
#39408=VERTEX_POINT ( 'NONE', #45044 ) ;
#39415=VECTOR ( 'NONE', #8123, 39.37007874015748854 ) ;
#39577=CARTESIAN_POINT ( 'NONE',  ( 0.1574803149606299191, 0.5360961046428496246, -0.7563373642699310340 ) ) ;
#39601=ADVANCED_FACE ( 'NONE', ( #12029 ), #25707, .F. ) ;
#39642=CARTESIAN_POINT ( 'NONE',  ( -1.707404996040165498E-16, 1.086379535891622172, -0.03715491745705901822 ) ) ;
#39654=EDGE_LOOP ( 'NONE', ( #13623, #12015, #14248, #44332 ) ) ;
#39730=ORIENTED_EDGE ( 'NONE', *, *, #36636, .F. ) ;
#39869=VECTOR ( 'NONE', #38029, 39.37007874015748143 ) ;
#39890=LINE ( 'NONE', #1526, #47253 ) ;
#39895=ORIENTED_EDGE ( 'NONE', *, *, #24562, .T. ) ;
#39918=DIRECTION ( 'NONE',  ( 2.943801717310650128E-16, -1.000000000000000000, -2.355041373848520102E-15 ) ) ;
#39921=ADVANCED_FACE ( 'NONE', ( #34962 ), #23035, .T. ) ;
#39976=DIRECTION ( 'NONE',  ( 0.000000000000000000, 1.000000000000000000, 0.000000000000000000 ) ) ;
#40068=CARTESIAN_POINT ( 'NONE',  ( 0.1864803149606299171, 0.5288907983920102529, -0.7507079620615728643 ) ) ;
#40077=ORIENTED_EDGE ( 'NONE', *, *, #20714, .T. ) ;
#40151=FACE_OUTER_BOUND ( 'NONE', #8900, .T. ) ;
#40183=ORIENTED_EDGE ( 'NONE', *, *, #44289, .T. ) ;
#40211=PLANE ( 'NONE',  #27889 ) ;
#40229=DIRECTION ( 'NONE',  ( 5.377642775528101993E-15, -1.000000000000000000, 0.000000000000000000 ) ) ;
#40237=DIRECTION ( 'NONE',  ( 0.000000000000000000, 0.000000000000000000, -1.000000000000000000 ) ) ;
#40255=LINE ( 'NONE', #18694, #1400 ) ;
#40274=CARTESIAN_POINT ( 'NONE',  ( 0.2759478392031617933, -0.09842519685039370636, 1.713085361781125915 ) ) ;
#40318=ORIENTED_EDGE ( 'NONE', *, *, #13085, .T. ) ;
#40344=LINE ( 'NONE', #29867, #13170 ) ;
#40364=ORIENTED_EDGE ( 'NONE', *, *, #27428, .F. ) ;
#40382=VECTOR ( 'NONE', #19731, 39.37007874015748143 ) ;
#40397=DIRECTION ( 'NONE',  ( 1.000000000000000000, 0.000000000000000000, 0.000000000000000000 ) ) ;
#40401=FACE_OUTER_BOUND ( 'NONE', #21039, .T. ) ;
#40407=CARTESIAN_POINT ( 'NONE',  ( -0.4405986714762811229, 0.2431096003418886098, -0.1899380364129106546 ) ) ;
#40434=DIRECTION ( 'NONE',  ( -1.000000000000000000, -5.372880794957870593E-15, 4.197754538034579871E-15 ) ) ;
#40441=EDGE_CURVE ( 'NONE', #21057, #35279, #41216, .T. ) ;
#40463=LINE ( 'NONE', #22507, #28896 ) ;
#40479=DIRECTION ( 'NONE',  ( -1.000000000000000000, 5.411399086424350389E-15, -4.275490733183370330E-15 ) ) ;
#40484=CARTESIAN_POINT ( 'NONE',  ( 0.1864803149606299171, 1.086379535891623949, -0.03715491745706165500 ) ) ;
#40547=EDGE_LOOP ( 'NONE', ( #14065, #25056, #8157, #7222 ) ) ;
#40554=LINE ( 'NONE', #18996, #43985 ) ;
#40562=EDGE_CURVE ( 'NONE', #31929, #36844, #1360, .T. ) ;
#40573=DIRECTION ( 'NONE',  ( -1.000000000000000000, 5.472378587457090550E-15, -4.275490733183370330E-15 ) ) ;
#40586=PRODUCT_DEFINITION_SHAPE ( 'NONE', 'NONE',  #20410 ) ;
#40602=DIRECTION ( 'NONE',  ( 2.943801717310650128E-16, -1.000000000000000000, -2.355041373848520102E-15 ) ) ;
#40667=VERTEX_POINT ( 'NONE', #5343 ) ;
#40670=SURFACE_SIDE_STYLE ('',( #7867 ) ) ;
#40723=VERTEX_POINT ( 'NONE', #30795 ) ;
#40733=LENGTH_MEASURE_WITH_UNIT ( LENGTH_MEASURE( 0.02539999999999999897 ), #29789 ) ;
#40746=AXIS2_PLACEMENT_3D ( 'NONE', #32159, #31460, #35051 ) ;
#40796=EDGE_CURVE ( 'NONE', #17791, #34943, #23575, .T. ) ;
#40872=FACE_OUTER_BOUND ( 'NONE', #30227, .T. ) ;
#40984=CIRCLE ( 'NONE', #44048, 0.4724409448818899238 ) ;
#41044=CARTESIAN_POINT ( 'NONE',  ( 0.08946752424252873981, -0.5708661417322835607, 1.224299699984019663 ) ) ;
#41064=ORIENTED_EDGE ( 'NONE', *, *, #7951, .F. ) ;
#41158=LINE ( 'NONE', #22506, #39415 ) ;
#41191=CIRCLE ( 'NONE', #16753, 0.5905511811023621549 ) ;
#41216=CIRCLE ( 'NONE', #31221, 0.1574803149606300579 ) ;
#41237=DIRECTION ( 'NONE',  ( 2.891205793294680298E-16, -1.000000000000000000, 0.000000000000000000 ) ) ;
#41241=ADVANCED_FACE ( 'NONE', ( #1322 ), #4924, .T. ) ;
#41297=EDGE_LOOP ( 'NONE', ( #30129, #6797, #28771, #31250 ) ) ;
#41312=APPLICATION_CONTEXT ( 'automotive_design' ) ;
#41449=CARTESIAN_POINT ( 'NONE',  ( 0.2383973256948878072, 0.3740157480314960647, 1.112073044918586717 ) ) ;
#41477=FACE_OUTER_BOUND ( 'NONE', #32528, .T. ) ;
#41525=CARTESIAN_POINT ( 'NONE',  ( 0.4736248074375835060, 1.205832402325950792, -1.129708666049259902 ) ) ;
#41591=DIRECTION ( 'NONE',  ( -7.051687499798870116E-15, -1.406820448837680035E-16, -1.000000000000000000 ) ) ;
#41620=FACE_BOUND ( 'NONE', #44252, .T. ) ;
#41636=ADVANCED_FACE ( 'NONE', ( #12060 ), #24258, .T. ) ;
#41680=DIRECTION ( 'NONE',  ( 0.000000000000000000, -1.000000000000000000, 0.000000000000000000 ) ) ;
#41683=EDGE_CURVE ( 'NONE', #30077, #8512, #42432, .T. ) ;
#41689=CIRCLE ( 'NONE', #21055, 0.7874015748031496509 ) ;
#41771=CARTESIAN_POINT ( 'NONE',  ( 0.04756641494945763188, -0.5708661417322835607, 1.120507485783946766 ) ) ;
#41775=EDGE_LOOP ( 'NONE', ( #24434, #24997, #32294, #34789 ) ) ;
#41783=ORIENTED_EDGE ( 'NONE', *, *, #35518, .F. ) ;
#41847=ORIENTED_EDGE ( 'NONE', *, *, #14520, .F. ) ;
#41863=DIRECTION ( 'NONE',  ( 0.000000000000000000, 1.000000000000000000, 0.000000000000000000 ) ) ;
#41906=EDGE_LOOP ( 'NONE', ( #6525, #36327, #1839, #3830 ) ) ;
#41933=DIRECTION ( 'NONE',  ( 2.943801717310650128E-16, -1.000000000000000000, -2.355041373848520102E-15 ) ) ;
#41946=FACE_OUTER_BOUND ( 'NONE', #3055, .T. ) ;
#41978=DIRECTION ( 'NONE',  ( 5.724375810226264544E-16, 0.6156614753256587358, 0.7880107536067215701 ) ) ;
#41989=VECTOR ( 'NONE', #29613, 39.37007874015748854 ) ;
#42018=EDGE_CURVE ( 'NONE', #36896, #42619, #12898, .T. ) ;
#42026=ORIENTED_EDGE ( 'NONE', *, *, #17805, .T. ) ;
#42027=ORIENTED_EDGE ( 'NONE', *, *, #33699, .T. ) ;
#42036=ORIENTED_EDGE ( 'NONE', *, *, #29054, .F. ) ;
#42087=DIRECTION ( 'NONE',  ( -1.000000000000000000, 0.000000000000000000, 0.000000000000000000 ) ) ;
#42101=ORIENTED_EDGE ( 'NONE', *, *, #4250, .F. ) ;
#42221=CARTESIAN_POINT ( 'NONE',  ( 0.1574803149606299191, 0.08719492171395729074, -0.5641677032617165022 ) ) ;
#42227=CARTESIAN_POINT ( 'NONE',  ( 0.3108999017613323090, 0.9251089822459547252, -1.060267534067256046 ) ) ;
#42234=EDGE_LOOP ( 'NONE', ( #38197, #21870, #20746, #9648 ) ) ;
#42256=CARTESIAN_POINT ( 'NONE',  ( 0.2759478392031617933, 0.3740157480314960647, 1.713085361781125915 ) ) ;
#42355=DIRECTION ( 'NONE',  ( 0.000000000000000000, 1.000000000000000000, 0.000000000000000000 ) ) ;
#42368=EDGE_LOOP ( 'NONE', ( #13571, #41847, #33759, #4416 ) ) ;
#42432=CIRCLE ( 'NONE', #38622, 0.02900000000000001882 ) ;
#42440=DIRECTION ( 'NONE',  ( -1.000000000000000000, -2.980860836206319941E-17, 2.307906111702434570E-17 ) ) ;
#42441=VERTEX_POINT ( 'NONE', #15553 ) ;
#42580=CARTESIAN_POINT ( 'NONE',  ( 0.3161444924769519216, 1.495705267341507883, -0.3569552279982051712 ) ) ;
#42608=LINE ( 'NONE', #31870, #14969 ) ;
#42616=EDGE_CURVE ( 'NONE', #8512, #36844, #34831, .T. ) ;
#42619=VERTEX_POINT ( 'NONE', #23560 ) ;
#42632=CARTESIAN_POINT ( 'NONE',  ( 0.04756641494945747922, 0.3740157480314960647, 1.120507485783946766 ) ) ;
#42688=DIRECTION ( 'NONE',  ( 5.392424630175478286E-15, -0.2432573283306889156, 0.9699617890481125881 ) ) ;
#42722=ORIENTED_EDGE ( 'NONE', *, *, #24896, .T. ) ;
#42783=CARTESIAN_POINT ( 'NONE',  ( 0.000000000000000000, 0.5360961046428496246, -0.7563373642699310340 ) ) ;
#42791=DIRECTION ( 'NONE',  ( 1.000000000000000000, 0.000000000000000000, 0.000000000000000000 ) ) ;
#42808=CARTESIAN_POINT ( 'NONE',  ( 0.000000000000000000, 0.6241017553149685870, 0.3240160679609070948 ) ) ;
#42810=VECTOR ( 'NONE', #44904, 39.37007874015748854 ) ;
#42831=VECTOR ( 'NONE', #10457, 39.37007874015748143 ) ;
#42837=CARTESIAN_POINT ( 'NONE',  ( 0.1574803149606299191, 0.000000000000000000, 0.000000000000000000 ) ) ;
#42868=AXIS2_PLACEMENT_3D ( 'NONE', #31284, #12368, #4663 ) ;
#42894=VERTEX_POINT ( 'NONE', #22075 ) ;
#42931=VERTEX_POINT ( 'NONE', #17533 ) ;
#42940=DIRECTION ( 'NONE',  ( -1.000000000000000000, 0.000000000000000000, 7.047314121155780399E-15 ) ) ;
#42962=CARTESIAN_POINT ( 'NONE',  ( 0.000000000000000000, -5.122214988120488358E-16, -8.878505979408856939E-16 ) ) ;
#43000=EDGE_LOOP ( 'NONE', ( #19227, #34033, #30520, #20940 ) ) ;
#43029=CARTESIAN_POINT ( 'NONE',  ( 0.03372458374097397904, 0.7769110883301575399, -0.6069894663860452289 ) ) ;
#43030=VERTEX_POINT ( 'NONE', #15852 ) ;
#43146=LINE ( 'NONE', #17295, #10907 ) ;
#43155=CARTESIAN_POINT ( 'NONE',  ( 0.000000000000000000, 0.4003652867858621955, 0.7276473417831970103 ) ) ;
#43213=CARTESIAN_POINT ( 'NONE',  ( 0.4736248074375818407, 1.488499961090669288, -0.3513258257898456138 ) ) ;
#43233=CYLINDRICAL_SURFACE ( 'NONE', #4755, 0.02900000000000048025 ) ;
#43245=ORIENTED_EDGE ( 'NONE', *, *, #13686, .F. ) ;
#43298=CARTESIAN_POINT ( 'NONE',  ( 0.1574803149606299191, 0.5288907983920094757, -0.7507079620615707549 ) ) ;
#43309=DIRECTION ( 'NONE',  ( 0.000000000000000000, 0.000000000000000000, -1.000000000000000000 ) ) ;
#43322=AXIS2_PLACEMENT_3D ( 'NONE', #4317, #18950, #36709 ) ;
#43411=ORIENTED_EDGE ( 'NONE', *, *, #7036, .T. ) ;
#43422=VERTEX_POINT ( 'NONE', #15201 ) ;
#43498=ORIENTED_EDGE ( 'NONE', *, *, #16570, .F. ) ;
#43569=ORIENTED_EDGE ( 'NONE', *, *, #26274, .F. ) ;
#43585=LINE ( 'NONE', #6930, #36060 ) ;
#43614=AXIS2_PLACEMENT_3D ( 'NONE', #40484, #19166, #943 ) ;
#43709=AXIS2_PLACEMENT_3D ( 'NONE', #36819, #29681, #33009 ) ;
#43742=ORIENTED_EDGE ( 'NONE', *, *, #42616, .T. ) ;
#43755=ORIENTED_EDGE ( 'NONE', *, *, #41683, .F. ) ;
#43803=DIRECTION ( 'NONE',  ( 0.000000000000000000, 0.000000000000000000, -1.000000000000000000 ) ) ;
#43922=ADVANCED_FACE ( 'NONE', ( #6746 ), #20897, .F. ) ;
#43926=FACE_OUTER_BOUND ( 'NONE', #25120, .T. ) ;
#43957=DIRECTION ( 'NONE',  ( 5.724375810226260600E-16, 0.6156614753256579586, 0.7880107536067221252 ) ) ;
#43976=VERTEX_POINT ( 'NONE', #42221 ) ;
#43985=VECTOR ( 'NONE', #4143, 39.37007874015748143 ) ;
#44003=DIRECTION ( 'NONE',  ( 0.000000000000000000, -2.197428715927215401E-15, 1.000000000000000000 ) ) ;
#44011=VECTOR ( 'NONE', #18180, 39.37007874015748854 ) ;
#44030=EDGE_CURVE ( 'NONE', #29781, #5626, #40984, .T. ) ;
#44048=AXIS2_PLACEMENT_3D ( 'NONE', #40274, #14432, #29569 ) ;
#44051=( LENGTH_UNIT ( ) NAMED_UNIT ( * ) SI_UNIT ( $, .METRE. ) ) ;
#44061=ORIENTED_EDGE ( 'NONE', *, *, #33199, .T. ) ;
#44067=CARTESIAN_POINT ( 'NONE',  ( 0.1574803149606299191, 0.6241017553149685870, 0.3240160679609070948 ) ) ;
#44069=CARTESIAN_POINT ( 'NONE',  ( 0.3161444924769527542, 1.025704337919492115, -1.138861239548320858 ) ) ;
#44078=CARTESIAN_POINT ( 'NONE',  ( 0.1184675242425320824, -0.09842519685039370636, 1.713085361781127913 ) ) ;
#44108=ORIENTED_EDGE ( 'NONE', *, *, #44030, .F. ) ;
#44149=VERTEX_POINT ( 'NONE', #20824 ) ;
#44252=EDGE_LOOP ( 'NONE', ( #20999, #36784 ) ) ;
#44289=EDGE_CURVE ( 'NONE', #28784, #31929, #36864, .T. ) ;
#44312=CARTESIAN_POINT ( 'NONE',  ( 0.2759478392031586291, 0.3740157480314960647, 1.224299699984019663 ) ) ;
#44327=CARTESIAN_POINT ( 'NONE',  ( 0.1574803149606299191, 0.000000000000000000, 0.000000000000000000 ) ) ;
#44332=ORIENTED_EDGE ( 'NONE', *, *, #34652, .T. ) ;
#44342=CARTESIAN_POINT ( 'NONE',  ( 0.1574803149606299191, 0.1473293504822035527, -0.9532488779249704836 ) ) ;
#44346=CARTESIAN_POINT ( 'NONE',  ( 0.1126279540338996077, -0.5708661417322835607, 1.206847064312610129 ) ) ;
#44348=EDGE_CURVE ( 'NONE', #580, #28644, #18181, .T. ) ;
#44369=ORIENTED_EDGE ( 'NONE', *, *, #40441, .F. ) ;
#44413=DIRECTION ( 'NONE',  ( 0.000000000000000000, -1.000000000000000000, 0.000000000000000000 ) ) ;
#44431=VECTOR ( 'NONE', #32971, 39.37007874015748143 ) ;
#44463=CARTESIAN_POINT ( 'NONE',  ( 0.3161444924769519216, 1.495705267341507883, -0.3569552279982047271 ) ) ;
#44469=FACE_OUTER_BOUND ( 'NONE', #19416, .T. ) ;
#44510=( NAMED_UNIT ( * ) SI_UNIT ( $, .STERADIAN. ) SOLID_ANGLE_UNIT ( ) ) ;
#44532=DIRECTION ( 'NONE',  ( -1.000000000000000000, 0.000000000000000000, 0.000000000000000000 ) ) ;
#44553=ORIENTED_EDGE ( 'NONE', *, *, #11792, .F. ) ;
#44566=VERTEX_POINT ( 'NONE', #4725 ) ;
#44642=DIRECTION ( 'NONE',  ( -1.000000000000000000, 0.000000000000000000, 7.049916206369740876E-15 ) ) ;
#44679=DIRECTION ( 'NONE',  ( 1.000000000000000000, 0.000000000000000000, 0.000000000000000000 ) ) ;
#44681=EDGE_CURVE ( 'NONE', #45189, #40667, #20761, .T. ) ;
#44690=COLOUR_RGB ( '', 0.31764706, 0.68627451, 0.89019608) ;
#44710=CARTESIAN_POINT ( 'NONE',  ( 0.4736248074375866701, -0.09842519685039370636, 1.713085361781129690 ) ) ;
#44793=AXIS2_PLACEMENT_3D ( 'NONE', #45087, #12549, #24026 ) ;
#44828=ADVANCED_FACE ( 'NONE', ( #24604 ), #45924, .F. ) ;
#44856=DIRECTION ( 'NONE',  ( -1.000000000000000000, 0.000000000000000000, -6.938893903907220489E-15 ) ) ;
#44882=DIRECTION ( 'NONE',  ( -1.000000000000000000, 0.000000000000000000, 6.123233995736769734E-17 ) ) ;
#44904=DIRECTION ( 'NONE',  ( 0.000000000000000000, -0.7880107536067212370, 0.6156614753256591799 ) ) ;
#44909=VERTEX_POINT ( 'NONE', #26033 ) ;
#44949=EDGE_CURVE ( 'NONE', #7704, #44149, #3493, .T. ) ;
#45044=CARTESIAN_POINT ( 'NONE',  ( 0.000000000000000000, -0.5708661417322835607, -6.991093932140394160E-17 ) ) ;
#45061=AXIS2_PLACEMENT_3D ( 'NONE', #18725, #6765, #14444 ) ;
#45068=CYLINDRICAL_SURFACE ( 'NONE', #25291, 0.2362204724409449064 ) ;
#45074=AXIS2_PLACEMENT_3D ( 'NONE', #9228, #17350, #38456 ) ;
#45087=CARTESIAN_POINT ( 'NONE',  ( 0.1574803149606299191, 0.1473293504822035527, -0.9532488779249704836 ) ) ;
#45147=EDGE_CURVE ( 'NONE', #42931, #21023, #5479, .T. ) ;
#45151=DIRECTION ( 'NONE',  ( -1.000000000000000000, 0.000000000000000000, 0.000000000000000000 ) ) ;
#45169=VECTOR ( 'NONE', #25877, 39.37007874015748143 ) ;
#45189=VERTEX_POINT ( 'NONE', #6626 ) ;
#45190=DIRECTION ( 'NONE',  ( 0.000000000000000000, 6.980778575359379259E-17, -1.000000000000000000 ) ) ;
#45212=EDGE_CURVE ( 'NONE', #44149, #32266, #13824, .T. ) ;
#45226=CARTESIAN_POINT ( 'NONE',  ( 0.1574803149606299191, -5.122214988120488358E-16, -8.878505979408856939E-16 ) ) ;
#45233=VECTOR ( 'NONE', #36710, 39.37007874015748854 ) ;
#45241=CIRCLE ( 'NONE', #38386, 0.3937007874015747699 ) ;
#45261=DIRECTION ( 'NONE',  ( -1.000000000000000000, 0.000000000000000000, 7.049916206369740876E-15 ) ) ;
#45291=LINE ( 'NONE', #27132, #5446 ) ;
#45309=CIRCLE ( 'NONE', #24673, 0.1864803149606299448 ) ;
#45328=DIRECTION ( 'NONE',  ( 0.000000000000000000, -1.000000000000000000, 0.000000000000000000 ) ) ;
#45380=ADVANCED_FACE ( 'NONE', ( #7572 ), #18592, .T. ) ;
#45434=LINE ( 'NONE', #27516, #39869 ) ;
#45464=EDGE_LOOP ( 'NONE', ( #1655, #46987 ) ) ;
#45470=DIRECTION ( 'NONE',  ( 5.392424630175478286E-15, -0.2432573283306889156, 0.9699617890481125881 ) ) ;
#45536=CARTESIAN_POINT ( 'NONE',  ( 0.08946752424252873981, -0.5708661417322835607, 1.224299699984019663 ) ) ;
#45616=CARTESIAN_POINT ( 'NONE',  ( 0.1574803149606299191, 0.5288907983920094757, -0.7507079620615707549 ) ) ;
#45702=PLANE ( 'NONE',  #8520 ) ;
#45755=DIRECTION ( 'NONE',  ( -1.000000000000000000, 0.000000000000000000, 7.047314121155780399E-15 ) ) ;
#45788=AXIS2_PLACEMENT_3D ( 'NONE', #15270, #25823, #26057 ) ;
#45862=DIRECTION ( 'NONE',  ( -2.696301922142131245E-30, 0.6156614753256592909, 0.7880107536067212370 ) ) ;
#45889=LINE ( 'NONE', #5403, #16005 ) ;
#45900=CARTESIAN_POINT ( 'NONE',  ( 0.3161444924769295506, 1.209494567139728360, -1.479906699140346449 ) ) ;
#45924=PLANE ( 'NONE',  #31058 ) ;
#45927=CARTESIAN_POINT ( 'NONE',  ( 0.3108999017613326976, 1.482597719745565090, -0.3467144894627433027 ) ) ;
#45930=DIRECTION ( 'NONE',  ( 0.000000000000000000, 0.7907053606985359195, -0.6121968903568508757 ) ) ;
#46031=ORIENTED_EDGE ( 'NONE', *, *, #45212, .T. ) ;
#46065=DIRECTION ( 'NONE',  ( 1.000000000000000000, -9.297927578135879519E-16, 0.000000000000000000 ) ) ;
#46106=ORIENTED_EDGE ( 'NONE', *, *, #19656, .F. ) ;
#46184=EDGE_CURVE ( 'NONE', #18361, #24385, #30532, .T. ) ;
#46185=CARTESIAN_POINT ( 'NONE',  ( 0.3161444924769275522, 1.975221432870720495, -0.9622519263226653186 ) ) ;
#46253=ORIENTED_EDGE ( 'NONE', *, *, #31671, .T. ) ;
#46289=DIRECTION ( 'NONE',  ( -5.464378949326941559E-15, -1.000000000000000000, 0.000000000000000000 ) ) ;
#46381=DIMENSIONAL_EXPONENTS ( 1.000000000000000000, 0.000000000000000000, 0.000000000000000000, 0.000000000000000000, 0.000000000000000000, 0.000000000000000000, 0.000000000000000000 ) ;
#46426=FACE_OUTER_BOUND ( 'NONE', #18644, .T. ) ;
#46503=DIRECTION ( 'NONE',  ( 1.000000000000000000, 0.000000000000000000, 0.000000000000000000 ) ) ;
#46548=CYLINDRICAL_SURFACE ( 'NONE', #27361, 0.7874015748031496509 ) ;
#46639=DIRECTION ( 'NONE',  ( 1.000000000000000000, -5.411399086424350389E-15, 4.275490733183370330E-15 ) ) ;
#46643=AXIS2_PLACEMENT_3D ( 'NONE', #44078, #25888, #29044 ) ;
#46685=CARTESIAN_POINT ( 'NONE',  ( 0.2759478392031606275, -0.09842519685039370636, 1.555605046820498050 ) ) ;
#46754=AXIS2_PLACEMENT_3D ( 'NONE', #45536, #41933, #5540 ) ;
#46802=AXIS2_PLACEMENT_3D ( 'NONE', #7300, #33437, #14731 ) ;
#46840=ORIENTED_EDGE ( 'NONE', *, *, #8935, .T. ) ;
#46873=CARTESIAN_POINT ( 'NONE',  ( 0.1574803149606299191, -0.5708661417322835607, -6.991093932140394160E-17 ) ) ;
#46899=LINE ( 'NONE', #6879, #30019 ) ;
#46957=DIRECTION ( 'NONE',  ( 0.000000000000000000, -0.7880107536067206819, 0.6156614753256598460 ) ) ;
#46970=ORIENTED_EDGE ( 'NONE', *, *, #18776, .F. ) ;
#46987=ORIENTED_EDGE ( 'NONE', *, *, #18826, .T. ) ;
#46993=ORIENTED_EDGE ( 'NONE', *, *, #23757, .T. ) ;
#46998=CIRCLE ( 'NONE', #307, 0.4724409448818896462 ) ;
#47069=CARTESIAN_POINT ( 'NONE',  ( 0.1864803149606299171, 0.5288907983920102529, -0.7507079620615728643 ) ) ;
#47080=EDGE_CURVE ( 'NONE', #34914, #8746, #33186, .T. ) ;
#47225=CIRCLE ( 'NONE', #20429, 0.07874015748031495954 ) ;
#47253=VECTOR ( 'NONE', #30811, 39.37007874015748854 ) ;
#47263=PLANE ( 'NONE',  #45061 ) ;
#47287=ORIENTED_EDGE ( 'NONE', *, *, #1075, .T. ) ;
#47293=ADVANCED_FACE ( 'NONE', ( #33891 ), #1013, .F. ) ;
#47295=EDGE_CURVE ( 'NONE', #42894, #34892, #45309, .T. ) ;
#47298=CARTESIAN_POINT ( 'NONE',  ( 0.1864803149606299171, 0.5288907983920102529, -0.7507079620615728643 ) ) ;
#47314=CARTESIAN_POINT ( 'NONE',  ( 0.3161444924769295506, 1.209494567139728360, -1.479906699140346449 ) ) ;
#47395=EDGE_CURVE ( 'NONE', #1767, #32266, #43146, .T. ) ;
#47419=AXIS2_PLACEMENT_3D ( 'NONE', #25173, #3827, #40237 ) ;
ENDSEC;
END-ISO-10303-21;
